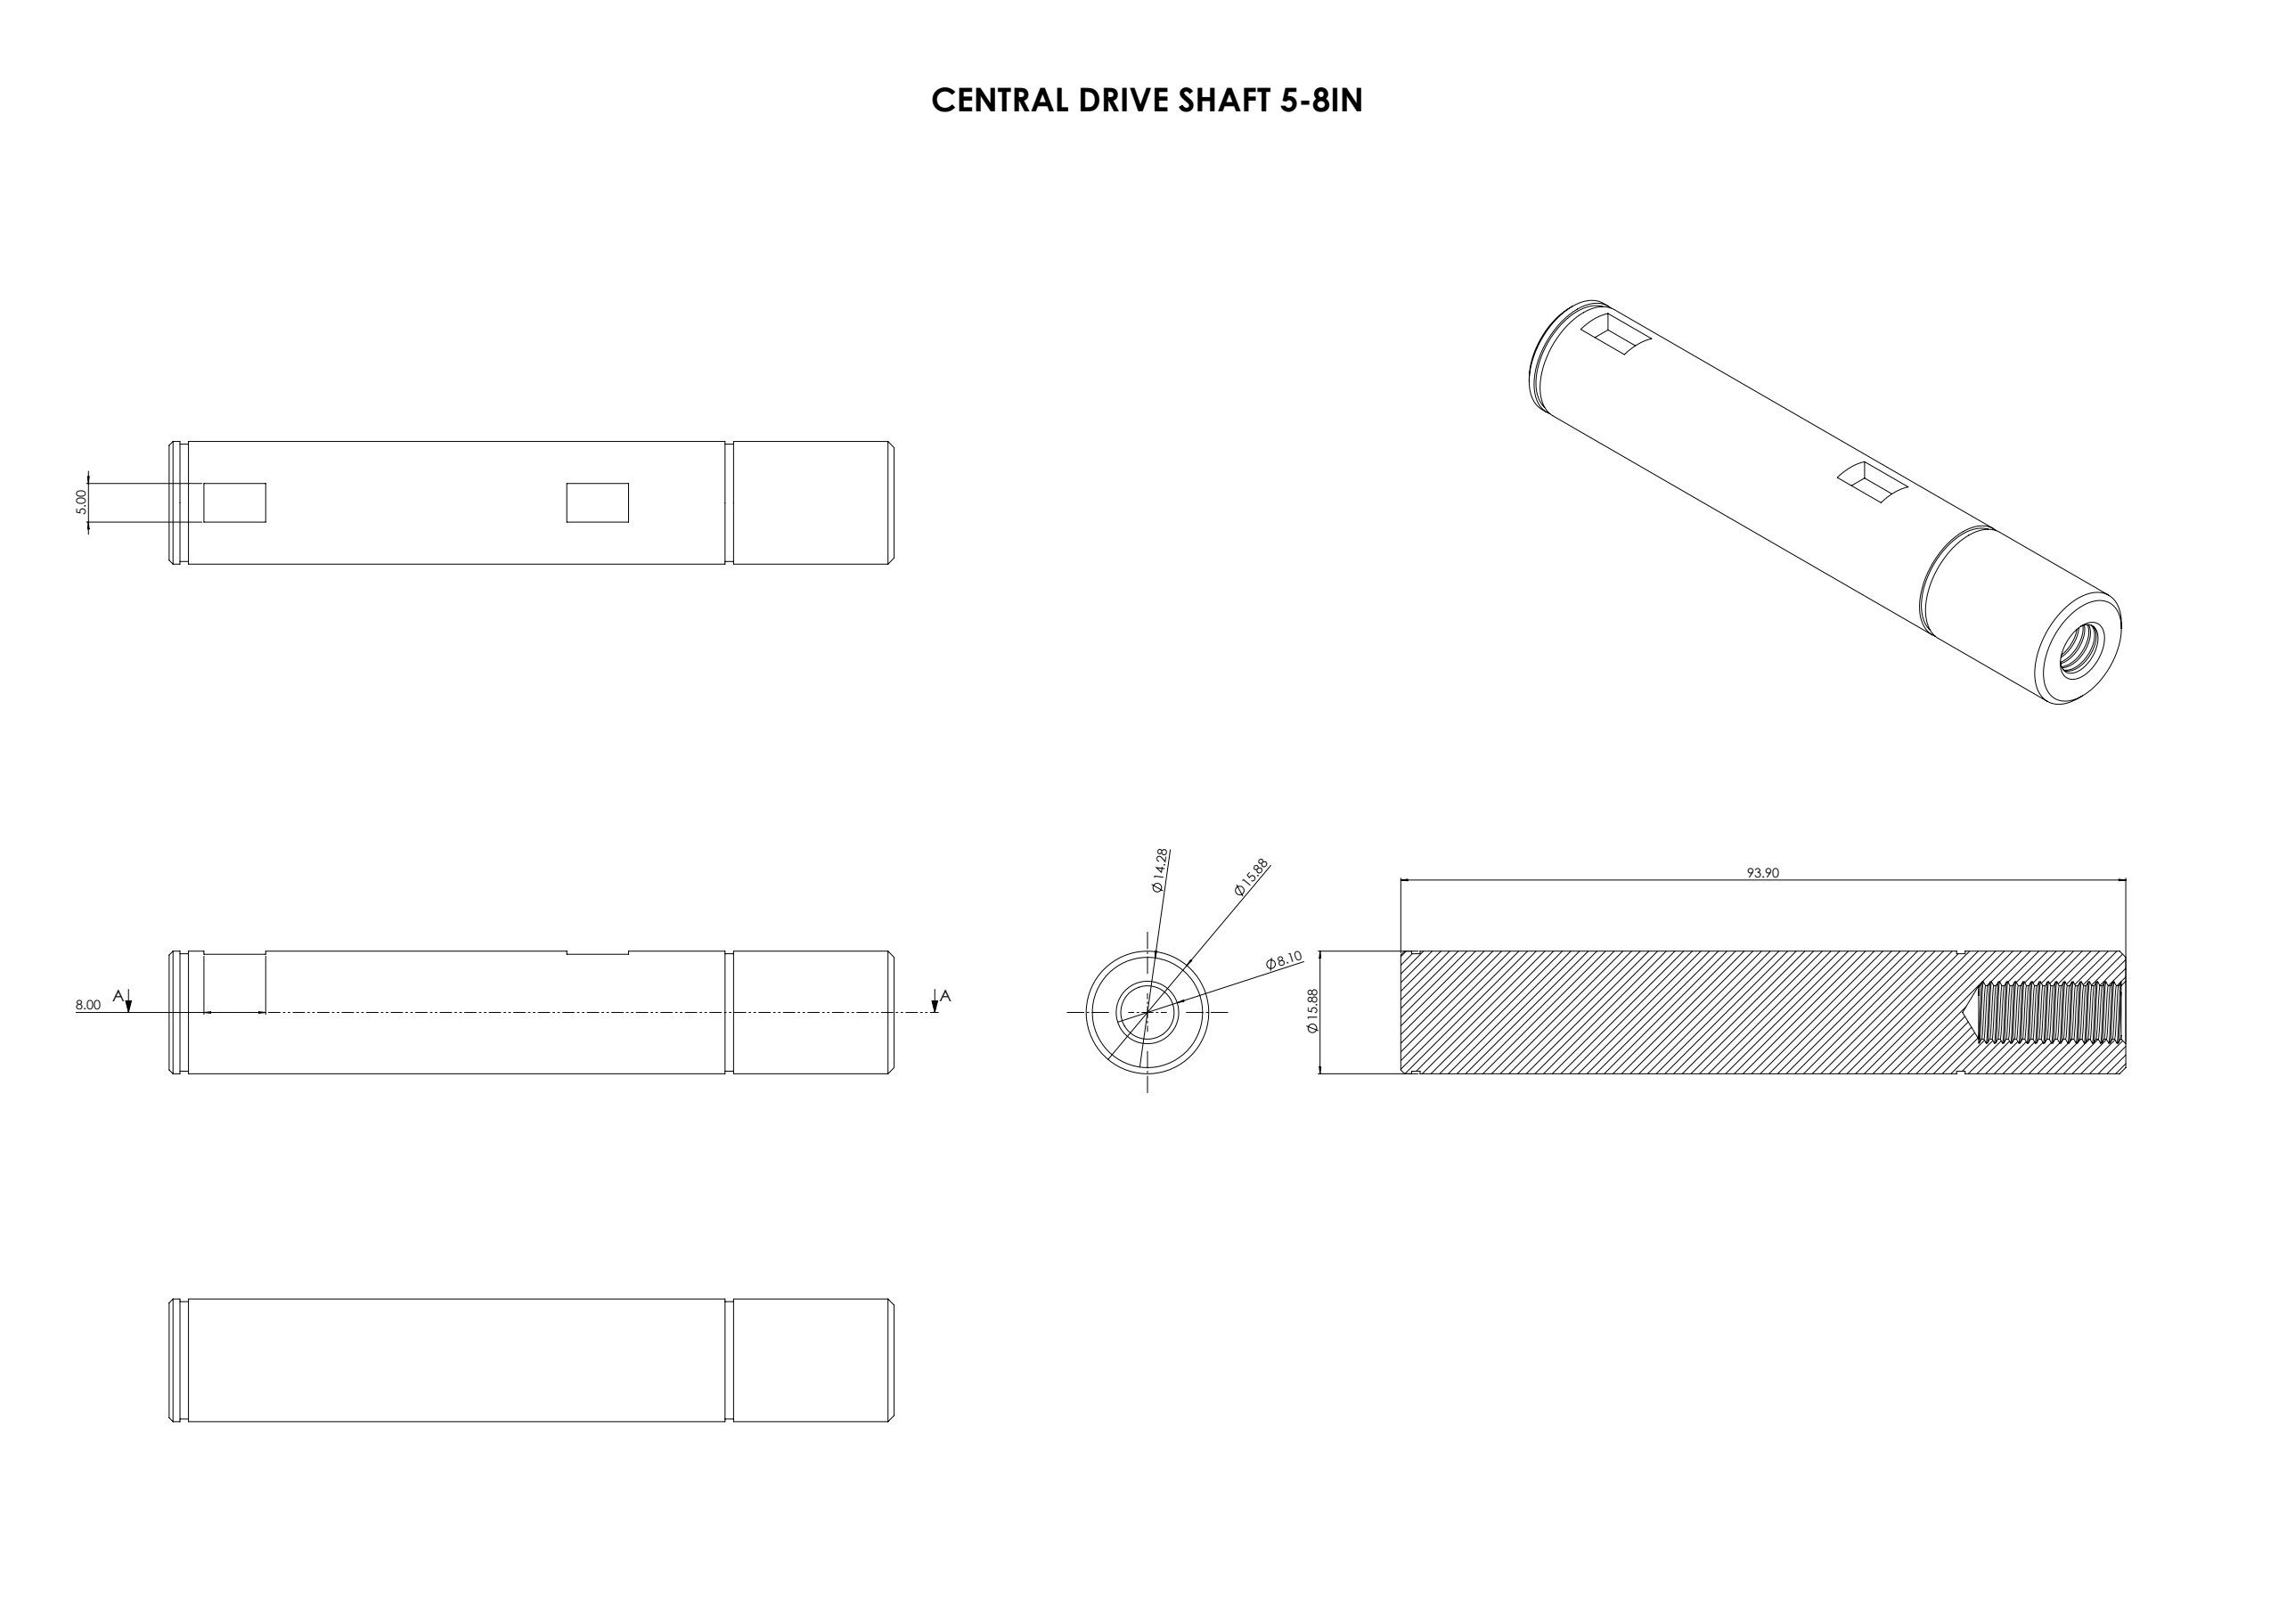
ISO-10303-21;
HEADER;
/* Generated by software containing ST-Developer
 * from STEP Tools, Inc. (www.steptools.com) 
 */

FILE_DESCRIPTION(
/* description */ (''),
/* implementation_level */ '2;1');

FILE_NAME(
/* name */ '03_Central_Drive_Shaft_5-8in.step',
/* time_stamp */ '2026-10-24T13:41:11-07:00',
/* author */ (''),
/* organization */ (''),
/* preprocessor_version */ 'ST-DEVELOPER v20.2',
/* originating_system */ 'Autodesk Translation Framework v15.15.0.0',
/* authorisation */ '');

FILE_SCHEMA (('AUTOMOTIVE_DESIGN { 1 0 10303 214 3 1 1 }'));
ENDSEC;

DATA;
#10=MECHANICAL_DESIGN_GEOMETRIC_PRESENTATION_REPRESENTATION('',(#123),#12813);
#85=CONICAL_SURFACE('',#4661,1.775,1.02974425867666);
#86=CONICAL_SURFACE('',#4663,3.85,0.785398163397459);
#87=CONICAL_SURFACE('',#4698,7.69,0.785398163397449);
#88=CONICAL_SURFACE('',#4701,7.54,0.785398163397436);
#103=SHAPE_REPRESENTATION_RELATIONSHIP('SRR','None',#12856,#113);
#113=ADVANCED_BREP_SHAPE_REPRESENTATION('',(#133),#12805);
#123=STYLED_ITEM('',(#12974),#133);
#133=MANIFOLD_SOLID_BREP('Body1',#4386);
#146=FACE_BOUND('',#701,.T.);
#147=FACE_BOUND('',#704,.T.);
#148=FACE_BOUND('',#706,.T.);
#149=FACE_BOUND('',#707,.T.);
#150=FACE_BOUND('',#709,.T.);
#151=FACE_BOUND('',#712,.T.);
#152=FACE_BOUND('',#719,.T.);
#178=PLANE('',#4654);
#179=PLANE('',#4658);
#180=PLANE('',#4665);
#181=PLANE('',#4666);
#182=PLANE('',#4668);
#183=PLANE('',#4669);
#184=PLANE('',#4671);
#185=PLANE('',#4672);
#186=PLANE('',#4673);
#187=PLANE('',#4675);
#188=PLANE('',#4676);
#189=PLANE('',#4678);
#190=PLANE('',#4679);
#191=PLANE('',#4684);
#192=PLANE('',#4688);
#193=PLANE('',#4692);
#194=PLANE('',#4696);
#195=PLANE('',#4703);
#306=B_SPLINE_SURFACE_WITH_KNOTS('',3,3,((#9182,#9183,#9184,#9185,#9186,
#9187,#9188,#9189,#9190,#9191,#9192,#9193,#9194,#9195,#9196,#9197,#9198,
#9199,#9200,#9201,#9202,#9203,#9204,#9205,#9206,#9207,#9208,#9209,#9210,
#9211,#9212,#9213,#9214,#9215,#9216,#9217,#9218,#9219,#9220,#9221,#9222,
#9223,#9224,#9225,#9226,#9227,#9228,#9229,#9230,#9231,#9232,#9233,#9234,
#9235,#9236,#9237,#9238,#9239,#9240,#9241,#9242,#9243,#9244,#9245,#9246,
#9247,#9248,#9249,#9250,#9251,#9252,#9253,#9254,#9255,#9256,#9257,#9258,
#9259,#9260,#9261,#9262,#9263,#9264,#9265,#9266,#9267,#9268,#9269,#9270,
#9271,#9272,#9273,#9274,#9275,#9276,#9277,#9278,#9279,#9280,#9281,#9282,
#9283,#9284,#9285,#9286,#9287,#9288,#9289,#9290,#9291,#9292,#9293,#9294,
#9295,#9296),(#9297,#9298,#9299,#9300,#9301,#9302,#9303,#9304,#9305,#9306,
#9307,#9308,#9309,#9310,#9311,#9312,#9313,#9314,#9315,#9316,#9317,#9318,
#9319,#9320,#9321,#9322,#9323,#9324,#9325,#9326,#9327,#9328,#9329,#9330,
#9331,#9332,#9333,#9334,#9335,#9336,#9337,#9338,#9339,#9340,#9341,#9342,
#9343,#9344,#9345,#9346,#9347,#9348,#9349,#9350,#9351,#9352,#9353,#9354,
#9355,#9356,#9357,#9358,#9359,#9360,#9361,#9362,#9363,#9364,#9365,#9366,
#9367,#9368,#9369,#9370,#9371,#9372,#9373,#9374,#9375,#9376,#9377,#9378,
#9379,#9380,#9381,#9382,#9383,#9384,#9385,#9386,#9387,#9388,#9389,#9390,
#9391,#9392,#9393,#9394,#9395,#9396,#9397,#9398,#9399,#9400,#9401,#9402,
#9403,#9404,#9405,#9406,#9407,#9408,#9409,#9410,#9411),(#9412,#9413,#9414,
#9415,#9416,#9417,#9418,#9419,#9420,#9421,#9422,#9423,#9424,#9425,#9426,
#9427,#9428,#9429,#9430,#9431,#9432,#9433,#9434,#9435,#9436,#9437,#9438,
#9439,#9440,#9441,#9442,#9443,#9444,#9445,#9446,#9447,#9448,#9449,#9450,
#9451,#9452,#9453,#9454,#9455,#9456,#9457,#9458,#9459,#9460,#9461,#9462,
#9463,#9464,#9465,#9466,#9467,#9468,#9469,#9470,#9471,#9472,#9473,#9474,
#9475,#9476,#9477,#9478,#9479,#9480,#9481,#9482,#9483,#9484,#9485,#9486,
#9487,#9488,#9489,#9490,#9491,#9492,#9493,#9494,#9495,#9496,#9497,#9498,
#9499,#9500,#9501,#9502,#9503,#9504,#9505,#9506,#9507,#9508,#9509,#9510,
#9511,#9512,#9513,#9514,#9515,#9516,#9517,#9518,#9519,#9520,#9521,#9522,
#9523,#9524,#9525,#9526),(#9527,#9528,#9529,#9530,#9531,#9532,#9533,#9534,
#9535,#9536,#9537,#9538,#9539,#9540,#9541,#9542,#9543,#9544,#9545,#9546,
#9547,#9548,#9549,#9550,#9551,#9552,#9553,#9554,#9555,#9556,#9557,#9558,
#9559,#9560,#9561,#9562,#9563,#9564,#9565,#9566,#9567,#9568,#9569,#9570,
#9571,#9572,#9573,#9574,#9575,#9576,#9577,#9578,#9579,#9580,#9581,#9582,
#9583,#9584,#9585,#9586,#9587,#9588,#9589,#9590,#9591,#9592,#9593,#9594,
#9595,#9596,#9597,#9598,#9599,#9600,#9601,#9602,#9603,#9604,#9605,#9606,
#9607,#9608,#9609,#9610,#9611,#9612,#9613,#9614,#9615,#9616,#9617,#9618,
#9619,#9620,#9621,#9622,#9623,#9624,#9625,#9626,#9627,#9628,#9629,#9630,
#9631,#9632,#9633,#9634,#9635,#9636,#9637,#9638,#9639,#9640,#9641)),
 .UNSPECIFIED.,.F.,.F.,.F.,(4,4),(4,1,1,1,1,1,1,1,1,1,1,1,1,1,1,1,1,1,1,
1,1,1,1,1,1,1,1,1,1,1,1,1,1,1,1,1,1,1,1,1,1,1,1,1,1,1,1,1,1,1,1,1,1,1,1,
1,1,1,1,1,1,1,1,1,1,1,1,1,1,1,1,1,1,1,1,1,1,1,1,1,1,1,1,1,1,1,1,1,1,1,1,
1,1,1,1,1,1,1,1,1,1,1,1,1,1,1,1,1,1,1,1,1,4),(0.,0.0593920221915367),(11.8785778954414,
12.8729398037614,13.8673017120813,14.8616636204013,15.8560255287213,16.8503874370412,
17.8447493453612,18.8391112536811,19.8334731620011,20.8278350703211,21.822196978641,
22.816558886961,23.810920795281,24.8052827036009,25.7996446119209,26.7940065202408,
27.7883684285608,28.7827303368808,29.7770922452007,30.7714541535207,31.7658160618407,
32.7601779701606,33.7545398784806,34.7489017868006,35.7432636951205,36.7376256034405,
37.7319875117605,38.7263494200804,39.7207113284004,40.7150732367203,41.7094351450403,
42.7037970533603,43.6981589616802,44.6925208700002,45.6868827783202,46.6812446866401,
47.6756065949601,48.6699685032801,49.6643304116,50.65869231992,51.6530542282399,
52.6474161365599,53.6417780448799,54.6361399531998,55.6305018615198,56.6248637698398,
57.6192256781597,58.6135875864797,59.6079494947996,60.6023114031196,61.5966733114396,
62.5910352197595,63.5853971280795,64.5797590363995,65.5741209447194,66.5684828530394,
67.5628447613594,68.5572066696793,69.5515685779993,70.5459304863193,71.5402923946392,
72.5346543029592,73.5290162112791,74.5233781195991,75.5177400279191,76.512101936239,
77.506463844559,78.500825752879,79.4951876611989,80.4895495695189,81.4839114778388,
82.4782733861588,83.4726352944788,84.4669972027987,85.4613591111187,86.4557210194387,
87.4500829277586,88.4444448360786,89.4388067443986,90.4331686527185,91.4275305610385,
92.4218924693585,93.4162543776784,94.4106162859984,95.4049781943183,96.3993401026383,
97.3937020109583,98.3880639192782,99.3824258275982,100.376787735918,101.371149644238,
102.365511552558,103.359873460878,104.354235369198,105.348597277518,106.342959185838,
107.337321094158,108.331683002478,109.326044910798,110.320406819118,111.314768727438,
112.309130635758,113.303492544078,114.297854452398,115.292216360718,116.286578269038,
117.280940177358,118.275302085678,119.269663993997,120.264025902317,121.258387810637,
122.252749718957,123.247111627277),.UNSPECIFIED.);
#307=B_SPLINE_SURFACE_WITH_KNOTS('',3,3,((#9835,#9836,#9837,#9838,#9839,
#9840,#9841,#9842,#9843,#9844,#9845,#9846,#9847,#9848,#9849,#9850,#9851,
#9852,#9853,#9854,#9855,#9856,#9857,#9858,#9859,#9860,#9861,#9862,#9863,
#9864,#9865,#9866,#9867,#9868,#9869,#9870,#9871,#9872,#9873,#9874,#9875,
#9876,#9877,#9878,#9879,#9880,#9881,#9882,#9883,#9884,#9885,#9886,#9887,
#9888,#9889,#9890,#9891,#9892,#9893,#9894,#9895,#9896,#9897,#9898,#9899,
#9900,#9901,#9902,#9903,#9904,#9905,#9906,#9907,#9908,#9909,#9910,#9911,
#9912,#9913,#9914,#9915,#9916,#9917,#9918,#9919,#9920,#9921,#9922,#9923,
#9924,#9925,#9926,#9927,#9928,#9929,#9930,#9931,#9932,#9933,#9934,#9935,
#9936,#9937,#9938,#9939,#9940,#9941,#9942,#9943,#9944,#9945,#9946,#9947,
#9948,#9949),(#9950,#9951,#9952,#9953,#9954,#9955,#9956,#9957,#9958,#9959,
#9960,#9961,#9962,#9963,#9964,#9965,#9966,#9967,#9968,#9969,#9970,#9971,
#9972,#9973,#9974,#9975,#9976,#9977,#9978,#9979,#9980,#9981,#9982,#9983,
#9984,#9985,#9986,#9987,#9988,#9989,#9990,#9991,#9992,#9993,#9994,#9995,
#9996,#9997,#9998,#9999,#10000,#10001,#10002,#10003,#10004,#10005,#10006,
#10007,#10008,#10009,#10010,#10011,#10012,#10013,#10014,#10015,#10016,#10017,
#10018,#10019,#10020,#10021,#10022,#10023,#10024,#10025,#10026,#10027,#10028,
#10029,#10030,#10031,#10032,#10033,#10034,#10035,#10036,#10037,#10038,#10039,
#10040,#10041,#10042,#10043,#10044,#10045,#10046,#10047,#10048,#10049,#10050,
#10051,#10052,#10053,#10054,#10055,#10056,#10057,#10058,#10059,#10060,#10061,
#10062,#10063,#10064),(#10065,#10066,#10067,#10068,#10069,#10070,#10071,
#10072,#10073,#10074,#10075,#10076,#10077,#10078,#10079,#10080,#10081,#10082,
#10083,#10084,#10085,#10086,#10087,#10088,#10089,#10090,#10091,#10092,#10093,
#10094,#10095,#10096,#10097,#10098,#10099,#10100,#10101,#10102,#10103,#10104,
#10105,#10106,#10107,#10108,#10109,#10110,#10111,#10112,#10113,#10114,#10115,
#10116,#10117,#10118,#10119,#10120,#10121,#10122,#10123,#10124,#10125,#10126,
#10127,#10128,#10129,#10130,#10131,#10132,#10133,#10134,#10135,#10136,#10137,
#10138,#10139,#10140,#10141,#10142,#10143,#10144,#10145,#10146,#10147,#10148,
#10149,#10150,#10151,#10152,#10153,#10154,#10155,#10156,#10157,#10158,#10159,
#10160,#10161,#10162,#10163,#10164,#10165,#10166,#10167,#10168,#10169,#10170,
#10171,#10172,#10173,#10174,#10175,#10176,#10177,#10178,#10179),(#10180,
#10181,#10182,#10183,#10184,#10185,#10186,#10187,#10188,#10189,#10190,#10191,
#10192,#10193,#10194,#10195,#10196,#10197,#10198,#10199,#10200,#10201,#10202,
#10203,#10204,#10205,#10206,#10207,#10208,#10209,#10210,#10211,#10212,#10213,
#10214,#10215,#10216,#10217,#10218,#10219,#10220,#10221,#10222,#10223,#10224,
#10225,#10226,#10227,#10228,#10229,#10230,#10231,#10232,#10233,#10234,#10235,
#10236,#10237,#10238,#10239,#10240,#10241,#10242,#10243,#10244,#10245,#10246,
#10247,#10248,#10249,#10250,#10251,#10252,#10253,#10254,#10255,#10256,#10257,
#10258,#10259,#10260,#10261,#10262,#10263,#10264,#10265,#10266,#10267,#10268,
#10269,#10270,#10271,#10272,#10273,#10274,#10275,#10276,#10277,#10278,#10279,
#10280,#10281,#10282,#10283,#10284,#10285,#10286,#10287,#10288,#10289,#10290,
#10291,#10292,#10293,#10294)),.UNSPECIFIED.,.F.,.F.,.F.,(4,4),(4,1,1,1,
1,1,1,1,1,1,1,1,1,1,1,1,1,1,1,1,1,1,1,1,1,1,1,1,1,1,1,1,1,1,1,1,1,1,1,1,
1,1,1,1,1,1,1,1,1,1,1,1,1,1,1,1,1,1,1,1,1,1,1,1,1,1,1,1,1,1,1,1,1,1,1,1,
1,1,1,1,1,1,1,1,1,1,1,1,1,1,1,1,1,1,1,1,1,1,1,1,1,1,1,1,1,1,1,1,1,1,1,1,
4),(0.,0.0593920221915367),(14.6327430048308,15.6271049131507,16.6214668214707,
17.6158287297907,18.6101906381106,19.6045525464306,20.5989144547506,21.5932763630705,
22.5876382713905,23.5820001797105,24.5763620880304,25.5707239963504,26.5650859046703,
27.5594478129903,28.5538097213103,29.5481716296302,30.5425335379502,31.5368954462702,
32.5312573545901,33.5256192629101,34.5199811712301,35.51434307955,36.50870498787,
37.5030668961899,38.4974288045099,39.4917907128299,40.4861526211498,41.4805145294698,
42.4748764377898,43.4692383461097,44.4636002544297,45.4579621627497,46.4523240710696,
47.4466859793896,48.4410478877095,49.4354097960295,50.4297717043495,51.4241336126694,
52.4184955209894,53.4128574293094,54.4072193376293,55.4015812459493,56.3959431542693,
57.3903050625892,58.3846669709092,59.3790288792291,60.3733907875491,61.3677526958691,
62.362114604189,63.356476512509,64.350838420829,65.3452003291489,66.3395622374689,
67.3339241457888,68.3282860541088,69.3226479624288,70.3170098707487,71.3113717790687,
72.3057336873887,73.3000955957086,74.2944575040286,75.2888194123486,76.2831813206685,
77.2775432289885,78.2719051373085,79.2662670456284,80.2606289539484,81.2549908622683,
82.2493527705883,83.2437146789083,84.2380765872282,85.2324384955482,86.2268004038682,
87.2211623121881,88.2155242205081,89.209886128828,90.204248037148,91.198609945468,
92.1929718537879,93.1873337621079,94.1816956704279,95.1760575787478,96.1704194870678,
97.1647813953878,98.1591433037077,99.1535052120277,100.147867120348,101.142229028668,
102.136590936988,103.130952845308,104.125314753628,105.119676661947,106.114038570267,
107.108400478587,108.102762386907,109.097124295227,110.091486203547,111.085848111867,
112.080210020187,113.074571928507,114.068933836827,115.063295745147,116.057657653467,
117.052019561787,118.046381470107,119.040743378427,120.035105286747,121.029467195067,
122.023829103387,123.018191011707,124.012552920027,125.006914828347,126.001276736667),
 .UNSPECIFIED.);
#372=FACE_OUTER_BOUND('',#647,.T.);
#373=FACE_OUTER_BOUND('',#648,.T.);
#374=FACE_OUTER_BOUND('',#649,.T.);
#375=FACE_OUTER_BOUND('',#650,.T.);
#376=FACE_OUTER_BOUND('',#651,.T.);
#377=FACE_OUTER_BOUND('',#652,.T.);
#378=FACE_OUTER_BOUND('',#653,.T.);
#379=FACE_OUTER_BOUND('',#654,.T.);
#380=FACE_OUTER_BOUND('',#655,.T.);
#381=FACE_OUTER_BOUND('',#656,.T.);
#382=FACE_OUTER_BOUND('',#657,.T.);
#383=FACE_OUTER_BOUND('',#658,.T.);
#384=FACE_OUTER_BOUND('',#659,.T.);
#385=FACE_OUTER_BOUND('',#660,.T.);
#386=FACE_OUTER_BOUND('',#661,.T.);
#387=FACE_OUTER_BOUND('',#662,.T.);
#388=FACE_OUTER_BOUND('',#663,.T.);
#389=FACE_OUTER_BOUND('',#664,.T.);
#390=FACE_OUTER_BOUND('',#665,.T.);
#391=FACE_OUTER_BOUND('',#666,.T.);
#392=FACE_OUTER_BOUND('',#667,.T.);
#393=FACE_OUTER_BOUND('',#668,.T.);
#394=FACE_OUTER_BOUND('',#669,.T.);
#395=FACE_OUTER_BOUND('',#670,.T.);
#396=FACE_OUTER_BOUND('',#671,.T.);
#397=FACE_OUTER_BOUND('',#672,.T.);
#398=FACE_OUTER_BOUND('',#673,.T.);
#399=FACE_OUTER_BOUND('',#674,.T.);
#400=FACE_OUTER_BOUND('',#675,.T.);
#401=FACE_OUTER_BOUND('',#676,.T.);
#402=FACE_OUTER_BOUND('',#677,.T.);
#403=FACE_OUTER_BOUND('',#678,.T.);
#404=FACE_OUTER_BOUND('',#679,.T.);
#405=FACE_OUTER_BOUND('',#680,.T.);
#406=FACE_OUTER_BOUND('',#681,.T.);
#407=FACE_OUTER_BOUND('',#682,.T.);
#408=FACE_OUTER_BOUND('',#683,.T.);
#409=FACE_OUTER_BOUND('',#684,.T.);
#410=FACE_OUTER_BOUND('',#685,.T.);
#411=FACE_OUTER_BOUND('',#686,.T.);
#412=FACE_OUTER_BOUND('',#687,.T.);
#413=FACE_OUTER_BOUND('',#688,.T.);
#414=FACE_OUTER_BOUND('',#689,.T.);
#415=FACE_OUTER_BOUND('',#690,.T.);
#416=FACE_OUTER_BOUND('',#691,.T.);
#417=FACE_OUTER_BOUND('',#692,.T.);
#418=FACE_OUTER_BOUND('',#693,.T.);
#419=FACE_OUTER_BOUND('',#694,.T.);
#420=FACE_OUTER_BOUND('',#695,.T.);
#421=FACE_OUTER_BOUND('',#696,.T.);
#422=FACE_OUTER_BOUND('',#697,.T.);
#423=FACE_OUTER_BOUND('',#698,.T.);
#424=FACE_OUTER_BOUND('',#699,.T.);
#425=FACE_OUTER_BOUND('',#700,.T.);
#426=FACE_OUTER_BOUND('',#702,.T.);
#427=FACE_OUTER_BOUND('',#703,.T.);
#428=FACE_OUTER_BOUND('',#705,.T.);
#429=FACE_OUTER_BOUND('',#708,.T.);
#430=FACE_OUTER_BOUND('',#710,.T.);
#431=FACE_OUTER_BOUND('',#711,.T.);
#432=FACE_OUTER_BOUND('',#713,.T.);
#433=FACE_OUTER_BOUND('',#714,.T.);
#434=FACE_OUTER_BOUND('',#715,.T.);
#435=FACE_OUTER_BOUND('',#716,.T.);
#436=FACE_OUTER_BOUND('',#717,.T.);
#437=FACE_OUTER_BOUND('',#718,.T.);
#647=EDGE_LOOP('',(#2997,#2998,#2999,#3000));
#648=EDGE_LOOP('',(#3001,#3002,#3003,#3004));
#649=EDGE_LOOP('',(#3005,#3006,#3007,#3008));
#650=EDGE_LOOP('',(#3009,#3010,#3011,#3012));
#651=EDGE_LOOP('',(#3013,#3014,#3015,#3016));
#652=EDGE_LOOP('',(#3017,#3018,#3019,#3020));
#653=EDGE_LOOP('',(#3021,#3022,#3023,#3024));
#654=EDGE_LOOP('',(#3025,#3026,#3027,#3028));
#655=EDGE_LOOP('',(#3029,#3030,#3031,#3032));
#656=EDGE_LOOP('',(#3033,#3034,#3035,#3036));
#657=EDGE_LOOP('',(#3037,#3038,#3039,#3040));
#658=EDGE_LOOP('',(#3041,#3042,#3043,#3044));
#659=EDGE_LOOP('',(#3045,#3046,#3047,#3048));
#660=EDGE_LOOP('',(#3049,#3050,#3051,#3052));
#661=EDGE_LOOP('',(#3053,#3054,#3055,#3056));
#662=EDGE_LOOP('',(#3057,#3058,#3059,#3060));
#663=EDGE_LOOP('',(#3061,#3062,#3063,#3064));
#664=EDGE_LOOP('',(#3065,#3066,#3067,#3068));
#665=EDGE_LOOP('',(#3069,#3070,#3071,#3072));
#666=EDGE_LOOP('',(#3073,#3074,#3075,#3076));
#667=EDGE_LOOP('',(#3077,#3078,#3079,#3080));
#668=EDGE_LOOP('',(#3081,#3082,#3083,#3084));
#669=EDGE_LOOP('',(#3085,#3086,#3087,#3088));
#670=EDGE_LOOP('',(#3089,#3090,#3091,#3092));
#671=EDGE_LOOP('',(#3093,#3094,#3095,#3096));
#672=EDGE_LOOP('',(#3097,#3098,#3099,#3100));
#673=EDGE_LOOP('',(#3101,#3102,#3103,#3104));
#674=EDGE_LOOP('',(#3105,#3106,#3107,#3108));
#675=EDGE_LOOP('',(#3109,#3110,#3111,#3112));
#676=EDGE_LOOP('',(#3113,#3114,#3115,#3116));
#677=EDGE_LOOP('',(#3117,#3118,#3119,#3120));
#678=EDGE_LOOP('',(#3121,#3122,#3123,#3124));
#679=EDGE_LOOP('',(#3125,#3126,#3127,#3128));
#680=EDGE_LOOP('',(#3129,#3130,#3131,#3132));
#681=EDGE_LOOP('',(#3133,#3134,#3135,#3136));
#682=EDGE_LOOP('',(#3137,#3138,#3139,#3140,#3141));
#683=EDGE_LOOP('',(#3142,#3143,#3144,#3145));
#684=EDGE_LOOP('',(#3146,#3147,#3148,#3149,#3150,#3151,#3152,#3153,#3154,
#3155,#3156,#3157,#3158,#3159,#3160,#3161,#3162,#3163,#3164,#3165,#3166,
#3167,#3168,#3169,#3170,#3171,#3172,#3173,#3174,#3175,#3176,#3177,#3178,
#3179,#3180,#3181,#3182,#3183,#3184));
#685=EDGE_LOOP('',(#3185,#3186,#3187,#3188,#3189));
#686=EDGE_LOOP('',(#3190,#3191,#3192,#3193,#3194,#3195,#3196,#3197,#3198,
#3199,#3200,#3201,#3202,#3203,#3204,#3205,#3206,#3207,#3208,#3209,#3210,
#3211,#3212,#3213,#3214,#3215,#3216,#3217,#3218,#3219,#3220,#3221,#3222,
#3223,#3224,#3225,#3226,#3227,#3228));
#687=EDGE_LOOP('',(#3229,#3230,#3231,#3232,#3233));
#688=EDGE_LOOP('',(#3234,#3235,#3236,#3237));
#689=EDGE_LOOP('',(#3238,#3239,#3240,#3241,#3242,#3243));
#690=EDGE_LOOP('',(#3244,#3245,#3246,#3247));
#691=EDGE_LOOP('',(#3248,#3249,#3250,#3251));
#692=EDGE_LOOP('',(#3252,#3253,#3254,#3255));
#693=EDGE_LOOP('',(#3256,#3257,#3258,#3259));
#694=EDGE_LOOP('',(#3260,#3261,#3262,#3263));
#695=EDGE_LOOP('',(#3264,#3265,#3266,#3267));
#696=EDGE_LOOP('',(#3268,#3269,#3270,#3271));
#697=EDGE_LOOP('',(#3272,#3273,#3274,#3275));
#698=EDGE_LOOP('',(#3276,#3277,#3278,#3279));
#699=EDGE_LOOP('',(#3280,#3281,#3282,#3283));
#700=EDGE_LOOP('',(#3284));
#701=EDGE_LOOP('',(#3285));
#702=EDGE_LOOP('',(#3286,#3287,#3288,#3289));
#703=EDGE_LOOP('',(#3290));
#704=EDGE_LOOP('',(#3291));
#705=EDGE_LOOP('',(#3292,#3293,#3294,#3295));
#706=EDGE_LOOP('',(#3296,#3297,#3298,#3299));
#707=EDGE_LOOP('',(#3300,#3301,#3302,#3303));
#708=EDGE_LOOP('',(#3304));
#709=EDGE_LOOP('',(#3305));
#710=EDGE_LOOP('',(#3306,#3307,#3308,#3309));
#711=EDGE_LOOP('',(#3310));
#712=EDGE_LOOP('',(#3311));
#713=EDGE_LOOP('',(#3312,#3313,#3314,#3315));
#714=EDGE_LOOP('',(#3316));
#715=EDGE_LOOP('',(#3317,#3318,#3319,#3320));
#716=EDGE_LOOP('',(#3321,#3322,#3323,#3324));
#717=EDGE_LOOP('',(#3325,#3326,#3327,#3328));
#718=EDGE_LOOP('',(#3329));
#719=EDGE_LOOP('',(#3330));
#960=CIRCLE('',#4616,3.4544);
#961=CIRCLE('',#4633,3.4544);
#962=CIRCLE('',#4635,3.96875);
#963=CIRCLE('',#4653,3.96875);
#964=CIRCLE('',#4655,3.4544);
#965=CIRCLE('',#4656,3.4544);
#966=CIRCLE('',#4659,3.4544);
#967=CIRCLE('',#4660,3.4544);
#968=CIRCLE('',#4664,4.05000000000002);
#969=CIRCLE('',#4667,7.94);
#970=CIRCLE('',#4670,7.94);
#971=CIRCLE('',#4674,7.94);
#972=CIRCLE('',#4677,7.94);
#973=CIRCLE('',#4680,7.94);
#974=CIRCLE('',#4681,7.6);
#975=CIRCLE('',#4683,7.6);
#976=CIRCLE('',#4685,7.94);
#977=CIRCLE('',#4687,7.94);
#978=CIRCLE('',#4689,7.6);
#979=CIRCLE('',#4691,7.6);
#980=CIRCLE('',#4693,7.94);
#981=CIRCLE('',#4695,7.94);
#982=CIRCLE('',#4697,7.44);
#983=CIRCLE('',#4700,7.94);
#984=CIRCLE('',#4702,7.14);
#1145=LINE('',#7735,#1375);
#1146=LINE('',#7777,#1376);
#1147=LINE('',#7825,#1377);
#1148=LINE('',#7876,#1378);
#1149=LINE('',#7927,#1379);
#1150=LINE('',#7975,#1380);
#1151=LINE('',#8026,#1381);
#1152=LINE('',#8074,#1382);
#1153=LINE('',#8125,#1383);
#1154=LINE('',#8176,#1384);
#1155=LINE('',#8224,#1385);
#1156=LINE('',#8275,#1386);
#1157=LINE('',#8326,#1387);
#1158=LINE('',#8374,#1388);
#1159=LINE('',#8425,#1389);
#1160=LINE('',#8473,#1390);
#1161=LINE('',#8524,#1391);
#1162=LINE('',#8566,#1392);
#1163=LINE('',#8583,#1393);
#1164=LINE('',#8608,#1394);
#1165=LINE('',#8633,#1395);
#1166=LINE('',#8657,#1396);
#1167=LINE('',#8682,#1397);
#1168=LINE('',#8707,#1398);
#1169=LINE('',#8731,#1399);
#1170=LINE('',#8755,#1400);
#1171=LINE('',#8781,#1401);
#1172=LINE('',#8805,#1402);
#1173=LINE('',#8829,#1403);
#1174=LINE('',#8855,#1404);
#1175=LINE('',#8879,#1405);
#1176=LINE('',#8903,#1406);
#1177=LINE('',#8928,#1407);
#1178=LINE('',#8953,#1408);
#1179=LINE('',#8977,#1409);
#1180=LINE('',#10319,#1410);
#1181=LINE('',#10323,#1411);
#1182=LINE('',#10328,#1412);
#1183=LINE('',#10330,#1413);
#1184=LINE('',#10332,#1414);
#1185=LINE('',#10333,#1415);
#1186=LINE('',#10338,#1416);
#1187=LINE('',#10339,#1417);
#1188=LINE('',#10342,#1418);
#1189=LINE('',#10344,#1419);
#1190=LINE('',#10345,#1420);
#1191=LINE('',#10348,#1421);
#1192=LINE('',#10353,#1422);
#1193=LINE('',#10355,#1423);
#1194=LINE('',#10357,#1424);
#1195=LINE('',#10358,#1425);
#1196=LINE('',#10363,#1426);
#1197=LINE('',#10364,#1427);
#1198=LINE('',#10367,#1428);
#1199=LINE('',#10369,#1429);
#1200=LINE('',#10370,#1430);
#1201=LINE('',#10373,#1431);
#1202=LINE('',#10383,#1432);
#1203=LINE('',#10389,#1433);
#1204=LINE('',#10397,#1434);
#1205=LINE('',#10403,#1435);
#1206=LINE('',#10409,#1436);
#1207=LINE('',#10413,#1437);
#1208=LINE('',#10417,#1438);
#1375=VECTOR('',#5248,3.55);
#1376=VECTOR('',#5253,3.55);
#1377=VECTOR('',#5256,3.55);
#1378=VECTOR('',#5259,3.55);
#1379=VECTOR('',#5262,3.55);
#1380=VECTOR('',#5265,3.55);
#1381=VECTOR('',#5268,3.55);
#1382=VECTOR('',#5271,3.55);
#1383=VECTOR('',#5274,3.55);
#1384=VECTOR('',#5277,3.55);
#1385=VECTOR('',#5280,3.55);
#1386=VECTOR('',#5283,3.55);
#1387=VECTOR('',#5286,3.55);
#1388=VECTOR('',#5289,3.55);
#1389=VECTOR('',#5292,3.55);
#1390=VECTOR('',#5295,3.55);
#1391=VECTOR('',#5298,3.55);
#1392=VECTOR('',#5303,3.96875);
#1393=VECTOR('',#5308,3.96875);
#1394=VECTOR('',#5311,3.96875);
#1395=VECTOR('',#5314,3.96875);
#1396=VECTOR('',#5317,3.96875);
#1397=VECTOR('',#5320,3.96875);
#1398=VECTOR('',#5323,3.96875);
#1399=VECTOR('',#5326,3.96875);
#1400=VECTOR('',#5329,3.96875);
#1401=VECTOR('',#5332,3.96875);
#1402=VECTOR('',#5335,3.96875);
#1403=VECTOR('',#5338,3.96875);
#1404=VECTOR('',#5341,3.96875);
#1405=VECTOR('',#5344,3.96875);
#1406=VECTOR('',#5347,3.96875);
#1407=VECTOR('',#5350,3.96875);
#1408=VECTOR('',#5353,3.96875);
#1409=VECTOR('',#5356,3.96875);
#1410=VECTOR('',#5375,1.775);
#1411=VECTOR('',#5380,3.85);
#1412=VECTOR('',#5385,10.);
#1413=VECTOR('',#5386,10.);
#1414=VECTOR('',#5387,10.);
#1415=VECTOR('',#5388,10.);
#1416=VECTOR('',#5393,10.);
#1417=VECTOR('',#5394,10.);
#1418=VECTOR('',#5397,10.);
#1419=VECTOR('',#5398,10.);
#1420=VECTOR('',#5399,10.);
#1421=VECTOR('',#5404,10.);
#1422=VECTOR('',#5409,10.);
#1423=VECTOR('',#5410,10.);
#1424=VECTOR('',#5411,10.);
#1425=VECTOR('',#5412,10.);
#1426=VECTOR('',#5417,10.);
#1427=VECTOR('',#5418,10.);
#1428=VECTOR('',#5421,10.);
#1429=VECTOR('',#5422,10.);
#1430=VECTOR('',#5423,10.);
#1431=VECTOR('',#5428,10.);
#1432=VECTOR('',#5441,7.6);
#1433=VECTOR('',#5448,7.94);
#1434=VECTOR('',#5459,7.6);
#1435=VECTOR('',#5466,7.94);
#1436=VECTOR('',#5475,7.69);
#1437=VECTOR('',#5480,7.94);
#1438=VECTOR('',#5485,7.54);
#1606=B_SPLINE_CURVE_WITH_KNOTS('',3,(#7737,#7738,#7739,#7740,#7741,#7742,
#7743,#7744,#7745,#7746,#7747,#7748,#7749),.UNSPECIFIED.,.F.,.F.,(4,3,3,
3,4),(107.889370485171,108.385448006876,109.379809915196,110.374171823516,
111.368533731836),.UNSPECIFIED.);
#1607=B_SPLINE_CURVE_WITH_KNOTS('',3,(#7752,#7753,#7754,#7755,#7756,#7757,
#7758,#7759,#7760,#7761,#7762,#7763,#7764,#7765,#7766,#7767,#7768,#7769,
#7770,#7771,#7772,#7773),.UNSPECIFIED.,.F.,.F.,(4,3,3,3,3,3,3,4),(-109.6055207498,
-109.379809915196,-108.385448006876,-107.391086098556,-106.396724190236,
-105.402362281916,-104.408000373596,-104.360350287381),.UNSPECIFIED.);
#1608=B_SPLINE_CURVE_WITH_KNOTS('',3,(#7778,#7779,#7780,#7781,#7782,#7783,
#7784,#7785,#7786,#7787,#7788,#7789,#7790,#7791,#7792,#7793,#7794,#7795,
#7796,#7797,#7798,#7799),.UNSPECIFIED.,.F.,.F.,(4,3,3,3,3,3,3,4),(101.606185177992,
102.419276556956,103.413638465276,104.408000373596,105.402362281916,106.396724190236,
107.391086098556,107.889370485171),.UNSPECIFIED.);
#1609=B_SPLINE_CURVE_WITH_KNOTS('',3,(#7800,#7801,#7802,#7803,#7804,#7805,
#7806,#7807,#7808,#7809,#7810,#7811,#7812,#7813,#7814,#7815,#7816,#7817,
#7818,#7819,#7820,#7821),.UNSPECIFIED.,.F.,.F.,(4,3,3,3,3,3,3,4),(-104.360350287381,
-103.413638465276,-102.419276556956,-101.424914648636,-100.430552740316,
-99.4361908319964,-98.4418289236764,-98.0771649802013),.UNSPECIFIED.);
#1610=B_SPLINE_CURVE_WITH_KNOTS('',3,(#7826,#7827,#7828,#7829,#7830,#7831,
#7832,#7833,#7834,#7835,#7836,#7837,#7838,#7839,#7840,#7841,#7842,#7843,
#7844,#7845,#7846,#7847,#7848,#7849,#7850),.UNSPECIFIED.,.F.,.F.,(4,3,3,
3,3,3,3,3,4),(95.3229998708118,95.4587431987165,96.4531051070365,97.4474670153564,
98.4418289236764,99.4361908319964,100.430552740316,101.424914648636,101.606185177992),
 .UNSPECIFIED.);
#1611=B_SPLINE_CURVE_WITH_KNOTS('',3,(#7851,#7852,#7853,#7854,#7855,#7856,
#7857,#7858,#7859,#7860,#7861,#7862,#7863,#7864,#7865,#7866,#7867,#7868,
#7869,#7870,#7871,#7872),.UNSPECIFIED.,.F.,.F.,(4,3,3,3,3,3,3,4),(-98.0771649802013,
-97.4474670153564,-96.4531051070365,-95.4587431987165,-94.4643812903965,
-93.4700193820766,-92.4756574737566,-91.7939796730218),.UNSPECIFIED.);
#1612=B_SPLINE_CURVE_WITH_KNOTS('',3,(#7877,#7878,#7879,#7880,#7881,#7882,
#7883,#7884,#7885,#7886,#7887,#7888,#7889,#7890,#7891,#7892,#7893,#7894,
#7895,#7896,#7897,#7898),.UNSPECIFIED.,.F.,.F.,(4,3,3,3,3,3,3,4),(89.0398145636323,
89.4925717487967,90.4869336571167,91.4812955654367,92.4756574737566,93.4700193820766,
94.4643812903965,95.3229998708118),.UNSPECIFIED.);
#1613=B_SPLINE_CURVE_WITH_KNOTS('',3,(#7899,#7900,#7901,#7902,#7903,#7904,
#7905,#7906,#7907,#7908,#7909,#7910,#7911,#7912,#7913,#7914,#7915,#7916,
#7917,#7918,#7919,#7920,#7921,#7922,#7923),.UNSPECIFIED.,.F.,.F.,(4,3,3,
3,3,3,3,3,4),(-91.7939796730218,-91.4812955654366,-90.4869336571167,-89.4925717487967,
-88.4982098404768,-87.5038479321568,-86.5094860238368,-85.5151241155169,
-85.5107943658422),.UNSPECIFIED.);
#1614=B_SPLINE_CURVE_WITH_KNOTS('',3,(#7928,#7929,#7930,#7931,#7932,#7933,
#7934,#7935,#7936,#7937,#7938,#7939,#7940,#7941,#7942,#7943,#7944,#7945,
#7946,#7947,#7948,#7949),.UNSPECIFIED.,.F.,.F.,(4,3,3,3,3,3,3,4),(82.7566292564527,
83.526400298877,84.5207622071969,85.5151241155169,86.5094860238368,87.5038479321568,
88.4982098404767,89.0398145636323),.UNSPECIFIED.);
#1615=B_SPLINE_CURVE_WITH_KNOTS('',3,(#7950,#7951,#7952,#7953,#7954,#7955,
#7956,#7957,#7958,#7959,#7960,#7961,#7962,#7963,#7964,#7965,#7966,#7967,
#7968,#7969,#7970,#7971),.UNSPECIFIED.,.F.,.F.,(4,3,3,3,3,3,3,4),(-85.5107943658422,
-84.5207622071969,-83.526400298877,-82.532038390557,-81.537676482237,-80.5433145739171,
-79.5489526655971,-79.2276090586625),.UNSPECIFIED.);
#1616=B_SPLINE_CURVE_WITH_KNOTS('',3,(#7976,#7977,#7978,#7979,#7980,#7981,
#7982,#7983,#7984,#7985,#7986,#7987,#7988,#7989,#7990,#7991,#7992,#7993,
#7994,#7995,#7996,#7997,#7998,#7999,#8000),.UNSPECIFIED.,.F.,.F.,(4,3,3,
3,3,3,3,3,4),(76.473443949273,76.5658669406372,77.5602288489572,78.5545907572771,
79.5489526655971,80.543314573917,81.537676482237,82.532038390557,82.7566292564527),
 .UNSPECIFIED.);
#1617=B_SPLINE_CURVE_WITH_KNOTS('',3,(#8001,#8002,#8003,#8004,#8005,#8006,
#8007,#8008,#8009,#8010,#8011,#8012,#8013,#8014,#8015,#8016,#8017,#8018,
#8019,#8020,#8021,#8022),.UNSPECIFIED.,.F.,.F.,(4,3,3,3,3,3,3,4),(-79.2276090586625,
-78.5545907572771,-77.5602288489572,-76.5658669406372,-75.5715050323172,
-74.5771431239973,-73.5827812156773,-72.944423751483),.UNSPECIFIED.);
#1618=B_SPLINE_CURVE_WITH_KNOTS('',3,(#8027,#8028,#8029,#8030,#8031,#8032,
#8033,#8034,#8035,#8036,#8037,#8038,#8039,#8040,#8041,#8042,#8043,#8044,
#8045,#8046,#8047,#8048),.UNSPECIFIED.,.F.,.F.,(4,3,3,3,3,3,3,4),(70.1902586420935,
70.5996954907174,71.5940573990374,72.5884193073573,73.5827812156773,74.5771431239973,
75.5715050323172,76.473443949273),.UNSPECIFIED.);
#1619=B_SPLINE_CURVE_WITH_KNOTS('',3,(#8049,#8050,#8051,#8052,#8053,#8054,
#8055,#8056,#8057,#8058,#8059,#8060,#8061,#8062,#8063,#8064,#8065,#8066,
#8067,#8068,#8069,#8070),.UNSPECIFIED.,.F.,.F.,(4,3,3,3,3,3,3,4),(-72.944423751483,
-72.5884193073574,-71.5940573990374,-70.5996954907174,-69.6053335823975,
-68.6109716740775,-67.6166097657575,-66.6612384443034),.UNSPECIFIED.);
#1620=B_SPLINE_CURVE_WITH_KNOTS('',3,(#8075,#8076,#8077,#8078,#8079,#8080,
#8081,#8082,#8083,#8084,#8085,#8086,#8087,#8088,#8089,#8090,#8091,#8092,
#8093,#8094,#8095,#8096),.UNSPECIFIED.,.F.,.F.,(4,3,3,3,3,3,3,4),(63.9070733349139,
64.6335240407976,65.6278859491176,66.6222478574375,67.6166097657575,68.6109716740775,
69.6053335823974,70.1902586420935),.UNSPECIFIED.);
#1621=B_SPLINE_CURVE_WITH_KNOTS('',3,(#8097,#8098,#8099,#8100,#8101,#8102,
#8103,#8104,#8105,#8106,#8107,#8108,#8109,#8110,#8111,#8112,#8113,#8114,
#8115,#8116,#8117,#8118,#8119,#8120,#8121),.UNSPECIFIED.,.F.,.F.,(4,3,3,
3,3,3,3,3,4),(-66.6612384443034,-66.6222478574376,-65.6278859491176,-64.6335240407977,
-63.6391621324777,-62.6448002241577,-61.6504383158378,-60.6560764075178,
-60.3780531371238),.UNSPECIFIED.);
#1622=B_SPLINE_CURVE_WITH_KNOTS('',3,(#8126,#8127,#8128,#8129,#8130,#8131,
#8132,#8133,#8134,#8135,#8136,#8137,#8138,#8139,#8140,#8141,#8142,#8143,
#8144,#8145,#8146,#8147,#8148,#8149,#8150),.UNSPECIFIED.,.F.,.F.,(4,3,3,
3,3,3,3,3,4),(57.6238880277343,57.6729906825579,58.6673525908779,59.6617144991978,
60.6560764075178,61.6504383158377,62.6448002241577,63.6391621324777,63.9070733349139),
 .UNSPECIFIED.);
#1623=B_SPLINE_CURVE_WITH_KNOTS('',3,(#8151,#8152,#8153,#8154,#8155,#8156,
#8157,#8158,#8159,#8160,#8161,#8162,#8163,#8164,#8165,#8166,#8167,#8168,
#8169,#8170,#8171,#8172),.UNSPECIFIED.,.F.,.F.,(4,3,3,3,3,3,3,4),(-60.3780531371238,
-59.6617144991978,-58.6673525908779,-57.6729906825579,-56.6786287742379,
-55.684266865918,-54.689904957598,-54.0948678299441),.UNSPECIFIED.);
#1624=B_SPLINE_CURVE_WITH_KNOTS('',3,(#8177,#8178,#8179,#8180,#8181,#8182,
#8183,#8184,#8185,#8186,#8187,#8188,#8189,#8190,#8191,#8192,#8193,#8194,
#8195,#8196,#8197,#8198),.UNSPECIFIED.,.F.,.F.,(4,3,3,3,3,3,3,4),(51.3407027205547,
51.7068192326381,52.7011811409581,53.695543049278,54.689904957598,55.684266865918,
56.6786287742379,57.6238880277343),.UNSPECIFIED.);
#1625=B_SPLINE_CURVE_WITH_KNOTS('',3,(#8199,#8200,#8201,#8202,#8203,#8204,
#8205,#8206,#8207,#8208,#8209,#8210,#8211,#8212,#8213,#8214,#8215,#8216,
#8217,#8218,#8219,#8220),.UNSPECIFIED.,.F.,.F.,(4,3,3,3,3,3,3,4),(-54.0948678299441,
-53.695543049278,-52.7011811409581,-51.7068192326381,-50.7124573243181,
-49.7180954159982,-48.7237335076782,-47.8116825227646),.UNSPECIFIED.);
#1626=B_SPLINE_CURVE_WITH_KNOTS('',3,(#8225,#8226,#8227,#8228,#8229,#8230,
#8231,#8232,#8233,#8234,#8235,#8236,#8237,#8238,#8239,#8240,#8241,#8242,
#8243,#8244,#8245,#8246),.UNSPECIFIED.,.F.,.F.,(4,3,3,3,3,3,3,4),(45.0575174133751,
45.7406477827183,46.7350096910383,47.7293715993583,48.7237335076782,49.7180954159982,
50.7124573243181,51.3407027205547),.UNSPECIFIED.);
#1627=B_SPLINE_CURVE_WITH_KNOTS('',3,(#8247,#8248,#8249,#8250,#8251,#8252,
#8253,#8254,#8255,#8256,#8257,#8258,#8259,#8260,#8261,#8262,#8263,#8264,
#8265,#8266,#8267,#8268,#8269,#8270,#8271),.UNSPECIFIED.,.F.,.F.,(4,3,3,
3,3,3,3,3,4),(-47.8116825227646,-47.7293715993582,-46.7350096910383,-45.7406477827183,
-44.7462858743984,-43.7519239660784,-42.7575620577584,-41.7632001494385,
-41.528497215585),.UNSPECIFIED.);
#1628=B_SPLINE_CURVE_WITH_KNOTS('',3,(#8276,#8277,#8278,#8279,#8280,#8281,
#8282,#8283,#8284,#8285,#8286,#8287,#8288,#8289,#8290,#8291,#8292,#8293,
#8294,#8295,#8296,#8297,#8298,#8299,#8300),.UNSPECIFIED.,.F.,.F.,(4,3,3,
3,3,3,3,3,4),(38.7743321061955,38.7801144244786,39.7744763327985,40.7688382411185,
41.7632001494385,42.7575620577584,43.7519239660784,44.7462858743984,45.0575174133751),
 .UNSPECIFIED.);
#1629=B_SPLINE_CURVE_WITH_KNOTS('',3,(#8301,#8302,#8303,#8304,#8305,#8306,
#8307,#8308,#8309,#8310,#8311,#8312,#8313,#8314,#8315,#8316,#8317,#8318,
#8319,#8320,#8321,#8322),.UNSPECIFIED.,.F.,.F.,(4,3,3,3,3,3,3,4),(-41.528497215585,
-40.7688382411185,-39.7744763327985,-38.7801144244786,-37.7857525161586,
-36.7913906078387,-35.7970286995187,-35.2453119084054),.UNSPECIFIED.);
#1630=B_SPLINE_CURVE_WITH_KNOTS('',3,(#8327,#8328,#8329,#8330,#8331,#8332,
#8333,#8334,#8335,#8336,#8337,#8338,#8339,#8340,#8341,#8342,#8343,#8344,
#8345,#8346,#8347,#8348),.UNSPECIFIED.,.F.,.F.,(4,3,3,3,3,3,3,4),(32.491146799016,
32.8139429745588,33.8083048828788,34.8026667911987,35.7970286995187,36.7913906078386,
37.7857525161586,38.7743321061955),.UNSPECIFIED.);
#1631=B_SPLINE_CURVE_WITH_KNOTS('',3,(#8349,#8350,#8351,#8352,#8353,#8354,
#8355,#8356,#8357,#8358,#8359,#8360,#8361,#8362,#8363,#8364,#8365,#8366,
#8367,#8368,#8369,#8370),.UNSPECIFIED.,.F.,.F.,(4,3,3,3,3,3,3,4),(-35.2453119084054,
-34.8026667911987,-33.8083048828788,-32.8139429745588,-31.8195810662388,
-30.8252191579189,-29.8308572495989,-28.9621266012258),.UNSPECIFIED.);
#1632=B_SPLINE_CURVE_WITH_KNOTS('',3,(#8375,#8376,#8377,#8378,#8379,#8380,
#8381,#8382,#8383,#8384,#8385,#8386,#8387,#8388,#8389,#8390,#8391,#8392,
#8393,#8394,#8395,#8396),.UNSPECIFIED.,.F.,.F.,(4,3,3,3,3,3,3,4),(26.2079614918363,
26.847771524639,27.842133432959,28.8364953412789,29.8308572495989,30.8252191579189,
31.8195810662388,32.491146799016),.UNSPECIFIED.);
#1633=B_SPLINE_CURVE_WITH_KNOTS('',3,(#8397,#8398,#8399,#8400,#8401,#8402,
#8403,#8404,#8405,#8406,#8407,#8408,#8409,#8410,#8411,#8412,#8413,#8414,
#8415,#8416,#8417,#8418,#8419,#8420,#8421),.UNSPECIFIED.,.F.,.F.,(4,3,3,
3,3,3,3,3,4),(-28.9621266012258,-28.836495341279,-27.842133432959,-26.847771524639,
-25.8534096163191,-24.8590477079991,-23.8646857996791,-22.8703238913592,
-22.6789412940462),.UNSPECIFIED.);
#1634=B_SPLINE_CURVE_WITH_KNOTS('',3,(#8426,#8427,#8428,#8429,#8430,#8431,
#8432,#8433,#8434,#8435,#8436,#8437,#8438,#8439,#8440,#8441,#8442,#8443,
#8444,#8445,#8446,#8447),.UNSPECIFIED.,.F.,.F.,(4,3,3,3,3,3,3,4),(19.9247761846567,
20.8816000747192,21.8759619830392,22.8703238913592,23.8646857996791,24.8590477079991,
25.8534096163191,26.2079614918363),.UNSPECIFIED.);
#1635=B_SPLINE_CURVE_WITH_KNOTS('',3,(#8448,#8449,#8450,#8451,#8452,#8453,
#8454,#8455,#8456,#8457,#8458,#8459,#8460,#8461,#8462,#8463,#8464,#8465,
#8466,#8467,#8468,#8469),.UNSPECIFIED.,.F.,.F.,(4,3,3,3,3,3,3,4),(-22.6789412940462,
-21.8759619830392,-20.8816000747192,-19.8872381663993,-18.8928762580793,
-17.8985143497593,-16.9041524414394,-16.3957559868666),.UNSPECIFIED.);
#1636=B_SPLINE_CURVE_WITH_KNOTS('',3,(#8474,#8475,#8476,#8477,#8478,#8479,
#8480,#8481,#8482,#8483,#8484,#8485,#8486,#8487,#8488,#8489,#8490,#8491,
#8492,#8493,#8494,#8495,#8496,#8497,#8498),.UNSPECIFIED.,.F.,.F.,(4,3,3,
3,3,3,3,3,4),(13.6415908774772,13.9210667164795,14.9154286247995,15.9097905331194,
16.9041524414394,17.8985143497593,18.8928762580793,19.8872381663993,19.9247761846567),
 .UNSPECIFIED.);
#1637=B_SPLINE_CURVE_WITH_KNOTS('',3,(#8499,#8500,#8501,#8502,#8503,#8504,
#8505,#8506,#8507,#8508,#8509,#8510,#8511,#8512,#8513,#8514,#8515,#8516,
#8517,#8518,#8519,#8520),.UNSPECIFIED.,.F.,.F.,(4,3,3,3,3,3,3,4),(-16.3957559868666,
-15.9097905331194,-14.9154286247995,-13.9210667164795,-12.9267048081595,
-11.9323428998396,-10.9379809915196,-10.1125706796871),.UNSPECIFIED.);
#1638=B_SPLINE_CURVE_WITH_KNOTS('',3,(#8526,#8527,#8528,#8529,#8530,#8531,
#8532,#8533,#8534,#8535,#8536,#8537,#8538),.UNSPECIFIED.,.F.,.F.,(4,3,3,
3,4),(-3.82938537250746,-2.98308572495989,-1.98872381663993,-0.994361908319963,
0.),.UNSPECIFIED.);
#1639=B_SPLINE_CURVE_WITH_KNOTS('',3,(#8541,#8542,#8543,#8544,#8545,#8546,
#8547,#8548,#8549,#8550,#8551,#8552,#8553,#8554,#8555,#8556,#8557,#8558,
#8559,#8560,#8561,#8562),.UNSPECIFIED.,.F.,.F.,(4,3,3,3,3,3,3,4),(1.76301298203565,
1.98872381663993,2.98308572495989,3.97744763327985,4.97180954159982,5.96617144991978,
6.96053335823975,7.35840557029759),.UNSPECIFIED.);
#1640=B_SPLINE_CURVE_WITH_KNOTS('',3,(#8568,#8569,#8570,#8571),
 .UNSPECIFIED.,.F.,.F.,(4,4),(122.522113490002,123.247111627277),
 .UNSPECIFIED.);
#1641=B_SPLINE_CURVE_WITH_KNOTS('',3,(#8574,#8575,#8576,#8577,#8578,#8579),
 .UNSPECIFIED.,.F.,.F.,(4,1,1,4),(122.522113490002,123.018191011707,124.012552920027,
124.238263754631),.UNSPECIFIED.);
#1642=B_SPLINE_CURVE_WITH_KNOTS('',3,(#8584,#8585,#8586,#8587,#8588,#8589,
#8590,#8591,#8592,#8593,#8594),.UNSPECIFIED.,.F.,.F.,(4,1,1,1,1,1,1,1,4),
(116.238928182822,116.286578269038,117.280940177358,118.275302085678,119.269663993997,
120.264025902317,121.258387810637,122.252749718957,122.522113490002),
 .UNSPECIFIED.);
#1643=B_SPLINE_CURVE_WITH_KNOTS('',3,(#8595,#8596,#8597,#8598,#8599,#8600,
#8601,#8602,#8603,#8604),.UNSPECIFIED.,.F.,.F.,(4,1,1,1,1,1,1,4),(116.238928182822,
117.052019561787,118.046381470107,119.040743378427,120.035105286747,121.029467195067,
122.023829103387,122.522113490002),.UNSPECIFIED.);
#1644=B_SPLINE_CURVE_WITH_KNOTS('',3,(#8609,#8610,#8611,#8612,#8613,#8614,
#8615,#8616,#8617,#8618),.UNSPECIFIED.,.F.,.F.,(4,1,1,1,1,1,1,4),(109.955742875643,
110.320406819118,111.314768727438,112.309130635758,113.303492544078,114.297854452398,
115.292216360718,116.238928182822),.UNSPECIFIED.);
#1645=B_SPLINE_CURVE_WITH_KNOTS('',3,(#8619,#8620,#8621,#8622,#8623,#8624,
#8625,#8626,#8627,#8628,#8629),.UNSPECIFIED.,.F.,.F.,(4,1,1,1,1,1,1,1,4),
(109.955742875643,110.091486203547,111.085848111867,112.080210020187,113.074571928507,
114.068933836827,115.063295745147,116.057657653467,116.238928182822),
 .UNSPECIFIED.);
#1646=B_SPLINE_CURVE_WITH_KNOTS('',3,(#8634,#8635,#8636,#8637,#8638,#8639,
#8640,#8641,#8642,#8643),.UNSPECIFIED.,.F.,.F.,(4,1,1,1,1,1,1,4),(103.672557568463,
104.354235369198,105.348597277518,106.342959185838,107.337321094158,108.331683002478,
109.326044910798,109.955742875643),.UNSPECIFIED.);
#1647=B_SPLINE_CURVE_WITH_KNOTS('',3,(#8644,#8645,#8646,#8647,#8648,#8649,
#8650,#8651,#8652,#8653),.UNSPECIFIED.,.F.,.F.,(4,1,1,1,1,1,1,4),(103.672557568463,
104.125314753628,105.119676661947,106.114038570267,107.108400478587,108.102762386907,
109.097124295227,109.955742875643),.UNSPECIFIED.);
#1648=B_SPLINE_CURVE_WITH_KNOTS('',3,(#8658,#8659,#8660,#8661,#8662,#8663,
#8664,#8665,#8666,#8667,#8668),.UNSPECIFIED.,.F.,.F.,(4,1,1,1,1,1,1,1,4),
(97.3893722612835,97.3937020109583,98.3880639192782,99.3824258275982,100.376787735918,
101.371149644238,102.365511552558,103.359873460878,103.672557568463),
 .UNSPECIFIED.);
#1649=B_SPLINE_CURVE_WITH_KNOTS('',3,(#8669,#8670,#8671,#8672,#8673,#8674,
#8675,#8676,#8677,#8678),.UNSPECIFIED.,.F.,.F.,(4,1,1,1,1,1,1,4),(97.3893722612835,
98.1591433037077,99.1535052120277,100.147867120348,101.142229028668,102.136590936988,
103.130952845308,103.672557568463),.UNSPECIFIED.);
#1650=B_SPLINE_CURVE_WITH_KNOTS('',3,(#8683,#8684,#8685,#8686,#8687,#8688,
#8689,#8690,#8691,#8692),.UNSPECIFIED.,.F.,.F.,(4,1,1,1,1,1,1,4),(91.106186954104,
91.4275305610385,92.4218924693585,93.4162543776784,94.4106162859984,95.4049781943183,
96.3993401026383,97.3893722612835),.UNSPECIFIED.);
#1651=B_SPLINE_CURVE_WITH_KNOTS('',3,(#8693,#8694,#8695,#8696,#8697,#8698,
#8699,#8700,#8701,#8702,#8703),.UNSPECIFIED.,.F.,.F.,(4,1,1,1,1,1,1,1,4),
(91.106186954104,91.198609945468,92.1929718537879,93.1873337621079,94.1816956704279,
95.1760575787478,96.1704194870678,97.1647813953878,97.3893722612835),
 .UNSPECIFIED.);
#1652=B_SPLINE_CURVE_WITH_KNOTS('',3,(#8708,#8709,#8710,#8711,#8712,#8713,
#8714,#8715,#8716,#8717),.UNSPECIFIED.,.F.,.F.,(4,1,1,1,1,1,1,4),(84.8230016469244,
85.4613591111187,86.4557210194387,87.4500829277586,88.4444448360786,89.4388067443986,
90.4331686527185,91.106186954104),.UNSPECIFIED.);
#1653=B_SPLINE_CURVE_WITH_KNOTS('',3,(#8718,#8719,#8720,#8721,#8722,#8723,
#8724,#8725,#8726,#8727),.UNSPECIFIED.,.F.,.F.,(4,1,1,1,1,1,1,4),(84.8230016469244,
85.2324384955482,86.2268004038682,87.2211623121881,88.2155242205081,89.209886128828,
90.204248037148,91.106186954104),.UNSPECIFIED.);
#1654=B_SPLINE_CURVE_WITH_KNOTS('',3,(#8732,#8733,#8734,#8735,#8736,#8737,
#8738,#8739,#8740,#8741),.UNSPECIFIED.,.F.,.F.,(4,1,1,1,1,1,1,4),(78.5398163397447,
79.4951876611989,80.4895495695189,81.4839114778388,82.4782733861588,83.4726352944788,
84.4669972027987,84.8230016469244),.UNSPECIFIED.);
#1655=B_SPLINE_CURVE_WITH_KNOTS('',3,(#8742,#8743,#8744,#8745,#8746,#8747,
#8748,#8749,#8750,#8751),.UNSPECIFIED.,.F.,.F.,(4,1,1,1,1,1,1,4),(78.5398163397447,
79.2662670456284,80.2606289539484,81.2549908622683,82.2493527705883,83.2437146789083,
84.2380765872282,84.8230016469244),.UNSPECIFIED.);
#1656=B_SPLINE_CURVE_WITH_KNOTS('',3,(#8756,#8757,#8758,#8759,#8760,#8761,
#8762,#8763,#8764,#8765,#8766),.UNSPECIFIED.,.F.,.F.,(4,1,1,1,1,1,1,1,4),
(72.2566310325652,72.5346543029592,73.5290162112791,74.5233781195991,75.5177400279191,
76.512101936239,77.506463844559,78.500825752879,78.5398163397447),
 .UNSPECIFIED.);
#1657=B_SPLINE_CURVE_WITH_KNOTS('',3,(#8767,#8768,#8769,#8770,#8771,#8772,
#8773,#8774,#8775,#8776,#8777),.UNSPECIFIED.,.F.,.F.,(4,1,1,1,1,1,1,1,4),
(72.2566310325652,72.3057336873887,73.3000955957086,74.2944575040286,75.2888194123486,
76.2831813206685,77.2775432289885,78.2719051373085,78.5398163397447),
 .UNSPECIFIED.);
#1658=B_SPLINE_CURVE_WITH_KNOTS('',3,(#8782,#8783,#8784,#8785,#8786,#8787,
#8788,#8789,#8790,#8791),.UNSPECIFIED.,.F.,.F.,(4,1,1,1,1,1,1,4),(65.9734457253856,
66.5684828530394,67.5628447613594,68.5572066696793,69.5515685779993,70.5459304863193,
71.5402923946392,72.2566310325652),.UNSPECIFIED.);
#1659=B_SPLINE_CURVE_WITH_KNOTS('',3,(#8792,#8793,#8794,#8795,#8796,#8797,
#8798,#8799,#8800,#8801),.UNSPECIFIED.,.F.,.F.,(4,1,1,1,1,1,1,4),(65.9734457253856,
66.3395622374689,67.3339241457888,68.3282860541088,69.3226479624288,70.3170098707487,
71.3113717790687,72.2566310325652),.UNSPECIFIED.);
#1660=B_SPLINE_CURVE_WITH_KNOTS('',3,(#8806,#8807,#8808,#8809,#8810,#8811,
#8812,#8813,#8814,#8815),.UNSPECIFIED.,.F.,.F.,(4,1,1,1,1,1,1,4),(59.690260418206,
60.6023114031196,61.5966733114396,62.5910352197595,63.5853971280795,64.5797590363995,
65.5741209447194,65.9734457253856),.UNSPECIFIED.);
#1661=B_SPLINE_CURVE_WITH_KNOTS('',3,(#8816,#8817,#8818,#8819,#8820,#8821,
#8822,#8823,#8824,#8825),.UNSPECIFIED.,.F.,.F.,(4,1,1,1,1,1,1,4),(59.690260418206,
60.3733907875491,61.3677526958691,62.362114604189,63.356476512509,64.350838420829,
65.3452003291489,65.9734457253856),.UNSPECIFIED.);
#1662=B_SPLINE_CURVE_WITH_KNOTS('',3,(#8830,#8831,#8832,#8833,#8834,#8835,
#8836,#8837,#8838,#8839,#8840),.UNSPECIFIED.,.F.,.F.,(4,1,1,1,1,1,1,1,4),
(53.4070751110264,53.6417780448799,54.6361399531998,55.6305018615198,56.6248637698398,
57.6192256781597,58.6135875864797,59.6079494947996,59.690260418206),
 .UNSPECIFIED.);
#1663=B_SPLINE_CURVE_WITH_KNOTS('',3,(#8841,#8842,#8843,#8844,#8845,#8846,
#8847,#8848,#8849,#8850,#8851),.UNSPECIFIED.,.F.,.F.,(4,1,1,1,1,1,1,1,4),
(53.4070751110264,53.4128574293094,54.4072193376293,55.4015812459493,56.3959431542693,
57.3903050625892,58.3846669709092,59.3790288792291,59.690260418206),
 .UNSPECIFIED.);
#1664=B_SPLINE_CURVE_WITH_KNOTS('',3,(#8856,#8857,#8858,#8859,#8860,#8861,
#8862,#8863,#8864,#8865),.UNSPECIFIED.,.F.,.F.,(4,1,1,1,1,1,1,4),(47.1238898038468,
47.6756065949601,48.6699685032801,49.6643304116,50.65869231992,51.6530542282399,
52.6474161365599,53.4070751110264),.UNSPECIFIED.);
#1665=B_SPLINE_CURVE_WITH_KNOTS('',3,(#8866,#8867,#8868,#8869,#8870,#8871,
#8872,#8873,#8874,#8875),.UNSPECIFIED.,.F.,.F.,(4,1,1,1,1,1,1,4),(47.1238898038468,
47.4466859793896,48.4410478877095,49.4354097960295,50.4297717043495,51.4241336126694,
52.4184955209894,53.4070751110264),.UNSPECIFIED.);
#1666=B_SPLINE_CURVE_WITH_KNOTS('',3,(#8880,#8881,#8882,#8883,#8884,#8885,
#8886,#8887,#8888,#8889),.UNSPECIFIED.,.F.,.F.,(4,1,1,1,1,1,1,4),(40.8407044966672,
41.7094351450403,42.7037970533603,43.6981589616802,44.6925208700002,45.6868827783202,
46.6812446866401,47.1238898038468),.UNSPECIFIED.);
#1667=B_SPLINE_CURVE_WITH_KNOTS('',3,(#8890,#8891,#8892,#8893,#8894,#8895,
#8896,#8897,#8898,#8899),.UNSPECIFIED.,.F.,.F.,(4,1,1,1,1,1,1,4),(40.8407044966672,
41.4805145294698,42.4748764377898,43.4692383461097,44.4636002544297,45.4579621627497,
46.4523240710696,47.1238898038468),.UNSPECIFIED.);
#1668=B_SPLINE_CURVE_WITH_KNOTS('',3,(#8904,#8905,#8906,#8907,#8908,#8909,
#8910,#8911,#8912,#8913,#8914),.UNSPECIFIED.,.F.,.F.,(4,1,1,1,1,1,1,1,4),
(34.5575191894876,34.7489017868006,35.7432636951205,36.7376256034405,37.7319875117605,
38.7263494200804,39.7207113284004,40.7150732367203,40.8407044966672),
 .UNSPECIFIED.);
#1669=B_SPLINE_CURVE_WITH_KNOTS('',3,(#8915,#8916,#8917,#8918,#8919,#8920,
#8921,#8922,#8923,#8924),.UNSPECIFIED.,.F.,.F.,(4,1,1,1,1,1,1,4),(34.5575191894876,
35.51434307955,36.50870498787,37.5030668961899,38.4974288045099,39.4917907128299,
40.4861526211498,40.8407044966672),.UNSPECIFIED.);
#1670=B_SPLINE_CURVE_WITH_KNOTS('',3,(#8929,#8930,#8931,#8932,#8933,#8934,
#8935,#8936,#8937,#8938),.UNSPECIFIED.,.F.,.F.,(4,1,1,1,1,1,1,4),(28.274333882308,
28.7827303368808,29.7770922452007,30.7714541535207,31.7658160618407,32.7601779701606,
33.7545398784806,34.5575191894876),.UNSPECIFIED.);
#1671=B_SPLINE_CURVE_WITH_KNOTS('',3,(#8939,#8940,#8941,#8942,#8943,#8944,
#8945,#8946,#8947,#8948,#8949),.UNSPECIFIED.,.F.,.F.,(4,1,1,1,1,1,1,1,4),
(28.274333882308,28.5538097213103,29.5481716296302,30.5425335379502,31.5368954462702,
32.5312573545901,33.5256192629101,34.5199811712301,34.5575191894876),
 .UNSPECIFIED.);
#1672=B_SPLINE_CURVE_WITH_KNOTS('',3,(#8954,#8955,#8956,#8957,#8958,#8959,
#8960,#8961,#8962,#8963),.UNSPECIFIED.,.F.,.F.,(4,1,1,1,1,1,1,4),(21.9911485751284,
22.816558886961,23.810920795281,24.8052827036009,25.7996446119209,26.7940065202408,
27.7883684285608,28.274333882308),.UNSPECIFIED.);
#1673=B_SPLINE_CURVE_WITH_KNOTS('',3,(#8964,#8965,#8966,#8967,#8968,#8969,
#8970,#8971,#8972,#8973),.UNSPECIFIED.,.F.,.F.,(4,1,1,1,1,1,1,4),(21.9911485751284,
22.5876382713905,23.5820001797105,24.5763620880304,25.5707239963504,26.5650859046703,
27.5594478129903,28.274333882308),.UNSPECIFIED.);
#1674=B_SPLINE_CURVE_WITH_KNOTS('',3,(#8979,#8980,#8981,#8982,#8983),
 .UNSPECIFIED.,.F.,.F.,(4,1,4),(14.6327430048308,15.6271049131507,15.7079632679489),
 .UNSPECIFIED.);
#1675=B_SPLINE_CURVE_WITH_KNOTS('',3,(#8986,#8987,#8988,#8989,#8990,#8991),
 .UNSPECIFIED.,.F.,.F.,(4,1,1,4),(13.6415908774771,13.8673017120813,14.8616636204013,
15.7079632679489),.UNSPECIFIED.);
#1676=B_SPLINE_CURVE_WITH_KNOTS('',3,(#8996,#8997,#8998,#8999,#9000,#9001,
#9002,#9003,#9004,#9005,#9006,#9007,#9008,#9009,#9010,#9011,#9012,#9013,
#9014,#9015,#9016,#9017,#9018,#9019,#9020,#9021,#9022,#9023,#9024,#9025,
#9026,#9027,#9028,#9029,#9030,#9031,#9032,#9033,#9034,#9035,#9036,#9037,
#9038,#9039,#9040,#9041,#9042,#9043,#9044,#9045,#9046,#9047,#9048,#9049,
#9050,#9051,#9052,#9053,#9054,#9055,#9056,#9057,#9058,#9059,#9060,#9061,
#9062,#9063,#9064,#9065,#9066,#9067,#9068,#9069,#9070,#9071,#9072,#9073,
#9074,#9075,#9076,#9077),.UNSPECIFIED.,.F.,.F.,(4,3,3,3,3,3,3,3,3,3,3,3,
3,3,3,3,3,3,3,3,3,3,3,3,3,3,3,4),(-0.659098020064273,-0.626583361418082,
-0.593277974374451,-0.55935451242369,-0.553527494448718,-0.547862782208884,
-0.513423105891954,-0.478559830537098,-0.456043474192613,-0.446497663053644,
-0.441032459037381,-0.405381589223341,-0.36977595468836,-0.334102467234791,
-0.316265723508006,-0.30668221639439,-0.301163149286353,-0.298428979781222,
-0.2643597751017,-0.228954386588656,-0.19290020592246,-0.168787680182153,
-0.157455049850378,-0.152068965805326,-0.114051724353995,-0.076872177317131,
-0.0384360886585655,0.),.UNSPECIFIED.);
#1677=B_SPLINE_CURVE_WITH_KNOTS('',3,(#9078,#9079,#9080,#9081,#9082,#9083,
#9084,#9085,#9086,#9087,#9088,#9089,#9090,#9091,#9092,#9093,#9094,#9095,
#9096,#9097,#9098,#9099,#9100,#9101,#9102,#9103,#9104,#9105,#9106,#9107,
#9108,#9109,#9110,#9111,#9112,#9113,#9114,#9115,#9116,#9117,#9118,#9119,
#9120,#9121,#9122,#9123,#9124,#9125,#9126,#9127,#9128,#9129,#9130,#9131,
#9132,#9133,#9134,#9135,#9136,#9137,#9138,#9139,#9140,#9141,#9142,#9143,
#9144,#9145,#9146,#9147,#9148,#9149,#9150,#9151,#9152,#9153,#9154,#9155,
#9156,#9157,#9158,#9159),.UNSPECIFIED.,.F.,.F.,(4,3,3,3,3,3,3,3,3,3,3,3,
3,3,3,3,3,3,3,3,3,3,3,3,3,3,3,4),(-0.657201022293968,-0.620843507912061,
-0.583812069642265,-0.545304753610891,-0.539298492849628,-0.533288478909317,
-0.49669576643024,-0.460284093722029,-0.437217774680684,-0.425131515458518,
-0.419071806367675,-0.383242240123574,-0.34808971350986,-0.311921627450565,
-0.293837584420918,-0.284384662265536,-0.278693413802068,-0.27575354139127,
-0.241284348717361,-0.206301309944578,-0.171212377127033,-0.149810829986154,
-0.13853214715148,-0.133449179146389,-0.0991640919442515,-0.0650684826066501,
-0.0318743752082536,0.),.UNSPECIFIED.);
#1678=B_SPLINE_CURVE_WITH_KNOTS('',3,(#9161,#9162,#9163,#9164,#9165,#9166,
#9167,#9168,#9169,#9170,#9171),.UNSPECIFIED.,.F.,.F.,(4,1,1,1,1,1,1,1,4),
(15.7079632679489,15.8560255287213,16.8503874370412,17.8447493453612,18.8391112536811,
19.8334731620011,20.8278350703211,21.822196978641,21.9911485751284),
 .UNSPECIFIED.);
#1679=B_SPLINE_CURVE_WITH_KNOTS('',3,(#9172,#9173,#9174,#9175,#9176,#9177,
#9178,#9179,#9180,#9181),.UNSPECIFIED.,.F.,.F.,(4,1,1,1,1,1,1,4),(15.7079632679489,
16.6214668214707,17.6158287297907,18.6101906381106,19.6045525464306,20.5989144547506,
21.5932763630705,21.9911485751284),.UNSPECIFIED.);
#1680=B_SPLINE_CURVE_WITH_KNOTS('',3,(#9642,#9643,#9644,#9645,#9646,#9647,
#9648,#9649,#9650,#9651,#9652,#9653,#9654,#9655,#9656,#9657,#9658,#9659,
#9660,#9661,#9662,#9663,#9664,#9665,#9666,#9667,#9668,#9669,#9670,#9671,
#9672,#9673,#9674,#9675,#9676,#9677,#9678,#9679,#9680,#9681,#9682,#9683,
#9684,#9685,#9686,#9687,#9688,#9689,#9690,#9691,#9692,#9693,#9694,#9695,
#9696,#9697,#9698,#9699,#9700,#9701,#9702,#9703,#9704,#9705,#9706,#9707,
#9708,#9709,#9710,#9711,#9712,#9713,#9714,#9715,#9716,#9717,#9718,#9719,
#9720,#9721,#9722,#9723),.UNSPECIFIED.,.F.,.F.,(4,3,3,3,3,3,3,3,3,3,3,3,
3,3,3,3,3,3,3,3,3,3,3,3,3,3,3,4),(-0.659098020064319,-0.626583355717508,
-0.593277963850765,-0.559354498782614,-0.553527466898513,-0.547862778460467,
-0.513423098595221,-0.478559821819824,-0.456043466564999,-0.446497640120997,
-0.441032457407506,-0.405381588000935,-0.369775954373192,-0.334102467077208,
-0.316265723429216,-0.306682216314082,-0.301163149097039,-0.298428979781224,
-0.264359779778512,-0.22895439423595,-0.192900215169359,-0.168787688273189,
-0.157455061634061,-0.152068971468546,-0.114051728601409,-0.0768721821854325,
-0.0384360910927163,0.),.UNSPECIFIED.);
#1681=B_SPLINE_CURVE_WITH_KNOTS('',3,(#9724,#9725,#9726,#9727,#9728,#9729,
#9730,#9731,#9732,#9733,#9734,#9735,#9736,#9737,#9738,#9739,#9740,#9741,
#9742,#9743,#9744,#9745,#9746,#9747,#9748),.UNSPECIFIED.,.F.,.F.,(4,3,3,
3,3,3,3,3,4),(-10.1125706796871,-9.94361908319964,-8.94925717487967,-7.95489526655971,
-6.96053335823974,-5.96617144991978,-4.97180954159982,-3.97744763327986,
-3.82938537250746),.UNSPECIFIED.);
#1682=B_SPLINE_CURVE_WITH_KNOTS('',3,(#9750,#9751,#9752,#9753,#9754,#9755,
#9756,#9757,#9758,#9759,#9760,#9761,#9762,#9763,#9764,#9765,#9766,#9767,
#9768,#9769,#9770,#9771,#9772,#9773,#9774,#9775,#9776,#9777,#9778,#9779,
#9780,#9781,#9782,#9783,#9784,#9785,#9786,#9787,#9788,#9789,#9790,#9791,
#9792,#9793,#9794,#9795,#9796,#9797,#9798,#9799,#9800,#9801,#9802,#9803,
#9804,#9805,#9806,#9807,#9808,#9809,#9810,#9811,#9812,#9813,#9814,#9815,
#9816,#9817,#9818,#9819,#9820,#9821,#9822,#9823,#9824,#9825,#9826,#9827,
#9828,#9829,#9830,#9831),.UNSPECIFIED.,.F.,.F.,(4,3,3,3,3,3,3,3,3,3,3,3,
3,3,3,3,3,3,3,3,3,3,3,3,3,3,3,4),(-0.657201022293926,-0.620843512226781,
-0.583812075977012,-0.545304759153794,-0.539298504171762,-0.533288480271845,
-0.496695767933232,-0.460284093901184,-0.437217774837445,-0.425131516019463,
-0.419071806729443,-0.3832422403949,-0.348089712058185,-0.311921626724727,
-0.293837584057999,-0.284384661973879,-0.278693413430814,-0.27575354139127,
-0.241284348717361,-0.206301309906783,-0.171212377154442,-0.149810830010137,
-0.138532146710759,-0.133449178888522,-0.0991640917928147,-0.0650684819880444,
-0.0318743724222816,0.),.UNSPECIFIED.);
#1683=B_SPLINE_CURVE_WITH_KNOTS('',3,(#10295,#10296,#10297,#10298,#10299,
#10300,#10301,#10302,#10303,#10304,#10305,#10306,#10307,#10308,#10309,#10310,
#10311,#10312,#10313,#10314,#10315,#10316),.UNSPECIFIED.,.F.,.F.,(4,3,3,
3,3,3,3,4),(7.35840557029759,7.95489526655971,8.94925717487967,9.94361908319964,
10.9379809915196,11.9323428998396,12.9267048081595,13.6415908774772),
 .UNSPECIFIED.);
#1817=VERTEX_POINT('',#7733);
#1818=VERTEX_POINT('',#7734);
#1819=VERTEX_POINT('',#7736);
#1820=VERTEX_POINT('',#7750);
#1821=VERTEX_POINT('',#7775);
#1822=VERTEX_POINT('',#7776);
#1823=VERTEX_POINT('',#7823);
#1824=VERTEX_POINT('',#7824);
#1825=VERTEX_POINT('',#7874);
#1826=VERTEX_POINT('',#7875);
#1827=VERTEX_POINT('',#7925);
#1828=VERTEX_POINT('',#7926);
#1829=VERTEX_POINT('',#7973);
#1830=VERTEX_POINT('',#7974);
#1831=VERTEX_POINT('',#8024);
#1832=VERTEX_POINT('',#8025);
#1833=VERTEX_POINT('',#8072);
#1834=VERTEX_POINT('',#8073);
#1835=VERTEX_POINT('',#8123);
#1836=VERTEX_POINT('',#8124);
#1837=VERTEX_POINT('',#8174);
#1838=VERTEX_POINT('',#8175);
#1839=VERTEX_POINT('',#8222);
#1840=VERTEX_POINT('',#8223);
#1841=VERTEX_POINT('',#8273);
#1842=VERTEX_POINT('',#8274);
#1843=VERTEX_POINT('',#8324);
#1844=VERTEX_POINT('',#8325);
#1845=VERTEX_POINT('',#8372);
#1846=VERTEX_POINT('',#8373);
#1847=VERTEX_POINT('',#8423);
#1848=VERTEX_POINT('',#8424);
#1849=VERTEX_POINT('',#8471);
#1850=VERTEX_POINT('',#8472);
#1851=VERTEX_POINT('',#8522);
#1852=VERTEX_POINT('',#8523);
#1853=VERTEX_POINT('',#8525);
#1854=VERTEX_POINT('',#8539);
#1855=VERTEX_POINT('',#8564);
#1856=VERTEX_POINT('',#8565);
#1857=VERTEX_POINT('',#8567);
#1858=VERTEX_POINT('',#8572);
#1859=VERTEX_POINT('',#8581);
#1860=VERTEX_POINT('',#8582);
#1861=VERTEX_POINT('',#8606);
#1862=VERTEX_POINT('',#8607);
#1863=VERTEX_POINT('',#8631);
#1864=VERTEX_POINT('',#8632);
#1865=VERTEX_POINT('',#8655);
#1866=VERTEX_POINT('',#8656);
#1867=VERTEX_POINT('',#8680);
#1868=VERTEX_POINT('',#8681);
#1869=VERTEX_POINT('',#8705);
#1870=VERTEX_POINT('',#8706);
#1871=VERTEX_POINT('',#8729);
#1872=VERTEX_POINT('',#8730);
#1873=VERTEX_POINT('',#8753);
#1874=VERTEX_POINT('',#8754);
#1875=VERTEX_POINT('',#8779);
#1876=VERTEX_POINT('',#8780);
#1877=VERTEX_POINT('',#8803);
#1878=VERTEX_POINT('',#8804);
#1879=VERTEX_POINT('',#8827);
#1880=VERTEX_POINT('',#8828);
#1881=VERTEX_POINT('',#8853);
#1882=VERTEX_POINT('',#8854);
#1883=VERTEX_POINT('',#8877);
#1884=VERTEX_POINT('',#8878);
#1885=VERTEX_POINT('',#8901);
#1886=VERTEX_POINT('',#8902);
#1887=VERTEX_POINT('',#8926);
#1888=VERTEX_POINT('',#8927);
#1889=VERTEX_POINT('',#8951);
#1890=VERTEX_POINT('',#8952);
#1891=VERTEX_POINT('',#8975);
#1892=VERTEX_POINT('',#8976);
#1893=VERTEX_POINT('',#8978);
#1894=VERTEX_POINT('',#8984);
#1895=VERTEX_POINT('',#8993);
#1896=VERTEX_POINT('',#9832);
#1897=VERTEX_POINT('',#10318);
#1898=VERTEX_POINT('',#10322);
#1899=VERTEX_POINT('',#10326);
#1900=VERTEX_POINT('',#10327);
#1901=VERTEX_POINT('',#10329);
#1902=VERTEX_POINT('',#10331);
#1903=VERTEX_POINT('',#10335);
#1904=VERTEX_POINT('',#10337);
#1905=VERTEX_POINT('',#10341);
#1906=VERTEX_POINT('',#10343);
#1907=VERTEX_POINT('',#10351);
#1908=VERTEX_POINT('',#10352);
#1909=VERTEX_POINT('',#10354);
#1910=VERTEX_POINT('',#10356);
#1911=VERTEX_POINT('',#10360);
#1912=VERTEX_POINT('',#10362);
#1913=VERTEX_POINT('',#10366);
#1914=VERTEX_POINT('',#10368);
#1915=VERTEX_POINT('',#10376);
#1916=VERTEX_POINT('',#10378);
#1917=VERTEX_POINT('',#10381);
#1918=VERTEX_POINT('',#10385);
#1919=VERTEX_POINT('',#10388);
#1920=VERTEX_POINT('',#10392);
#1921=VERTEX_POINT('',#10395);
#1922=VERTEX_POINT('',#10399);
#1923=VERTEX_POINT('',#10402);
#1924=VERTEX_POINT('',#10406);
#1925=VERTEX_POINT('',#10411);
#1926=VERTEX_POINT('',#10415);
#2251=EDGE_CURVE('',#1817,#1818,#1145,.T.);
#2252=EDGE_CURVE('',#1818,#1819,#1606,.T.);
#2253=EDGE_CURVE('',#1819,#1820,#960,.T.);
#2254=EDGE_CURVE('',#1820,#1817,#1607,.T.);
#2255=EDGE_CURVE('',#1821,#1822,#1146,.T.);
#2256=EDGE_CURVE('',#1822,#1818,#1608,.T.);
#2257=EDGE_CURVE('',#1817,#1821,#1609,.T.);
#2258=EDGE_CURVE('',#1823,#1824,#1147,.T.);
#2259=EDGE_CURVE('',#1824,#1822,#1610,.T.);
#2260=EDGE_CURVE('',#1821,#1823,#1611,.T.);
#2261=EDGE_CURVE('',#1825,#1826,#1148,.T.);
#2262=EDGE_CURVE('',#1826,#1824,#1612,.T.);
#2263=EDGE_CURVE('',#1823,#1825,#1613,.T.);
#2264=EDGE_CURVE('',#1827,#1828,#1149,.T.);
#2265=EDGE_CURVE('',#1828,#1826,#1614,.T.);
#2266=EDGE_CURVE('',#1825,#1827,#1615,.T.);
#2267=EDGE_CURVE('',#1829,#1830,#1150,.T.);
#2268=EDGE_CURVE('',#1830,#1828,#1616,.T.);
#2269=EDGE_CURVE('',#1827,#1829,#1617,.T.);
#2270=EDGE_CURVE('',#1831,#1832,#1151,.T.);
#2271=EDGE_CURVE('',#1832,#1830,#1618,.T.);
#2272=EDGE_CURVE('',#1829,#1831,#1619,.T.);
#2273=EDGE_CURVE('',#1833,#1834,#1152,.T.);
#2274=EDGE_CURVE('',#1834,#1832,#1620,.T.);
#2275=EDGE_CURVE('',#1831,#1833,#1621,.T.);
#2276=EDGE_CURVE('',#1835,#1836,#1153,.T.);
#2277=EDGE_CURVE('',#1836,#1834,#1622,.T.);
#2278=EDGE_CURVE('',#1833,#1835,#1623,.T.);
#2279=EDGE_CURVE('',#1837,#1838,#1154,.T.);
#2280=EDGE_CURVE('',#1838,#1836,#1624,.T.);
#2281=EDGE_CURVE('',#1835,#1837,#1625,.T.);
#2282=EDGE_CURVE('',#1839,#1840,#1155,.T.);
#2283=EDGE_CURVE('',#1840,#1838,#1626,.T.);
#2284=EDGE_CURVE('',#1837,#1839,#1627,.T.);
#2285=EDGE_CURVE('',#1841,#1842,#1156,.T.);
#2286=EDGE_CURVE('',#1842,#1840,#1628,.T.);
#2287=EDGE_CURVE('',#1839,#1841,#1629,.T.);
#2288=EDGE_CURVE('',#1843,#1844,#1157,.T.);
#2289=EDGE_CURVE('',#1844,#1842,#1630,.T.);
#2290=EDGE_CURVE('',#1841,#1843,#1631,.T.);
#2291=EDGE_CURVE('',#1845,#1846,#1158,.T.);
#2292=EDGE_CURVE('',#1846,#1844,#1632,.T.);
#2293=EDGE_CURVE('',#1843,#1845,#1633,.T.);
#2294=EDGE_CURVE('',#1847,#1848,#1159,.T.);
#2295=EDGE_CURVE('',#1848,#1846,#1634,.T.);
#2296=EDGE_CURVE('',#1845,#1847,#1635,.T.);
#2297=EDGE_CURVE('',#1849,#1850,#1160,.T.);
#2298=EDGE_CURVE('',#1850,#1848,#1636,.T.);
#2299=EDGE_CURVE('',#1847,#1849,#1637,.T.);
#2300=EDGE_CURVE('',#1851,#1852,#1161,.T.);
#2301=EDGE_CURVE('',#1851,#1853,#1638,.T.);
#2302=EDGE_CURVE('',#1854,#1853,#961,.T.);
#2303=EDGE_CURVE('',#1854,#1852,#1639,.T.);
#2304=EDGE_CURVE('',#1855,#1856,#1162,.T.);
#2305=EDGE_CURVE('',#1856,#1857,#1640,.T.);
#2306=EDGE_CURVE('',#1858,#1857,#962,.T.);
#2307=EDGE_CURVE('',#1855,#1858,#1641,.T.);
#2308=EDGE_CURVE('',#1859,#1860,#1163,.T.);
#2309=EDGE_CURVE('',#1860,#1856,#1642,.T.);
#2310=EDGE_CURVE('',#1859,#1855,#1643,.T.);
#2311=EDGE_CURVE('',#1861,#1862,#1164,.T.);
#2312=EDGE_CURVE('',#1862,#1860,#1644,.T.);
#2313=EDGE_CURVE('',#1861,#1859,#1645,.T.);
#2314=EDGE_CURVE('',#1863,#1864,#1165,.T.);
#2315=EDGE_CURVE('',#1864,#1862,#1646,.T.);
#2316=EDGE_CURVE('',#1863,#1861,#1647,.T.);
#2317=EDGE_CURVE('',#1865,#1866,#1166,.T.);
#2318=EDGE_CURVE('',#1866,#1864,#1648,.T.);
#2319=EDGE_CURVE('',#1865,#1863,#1649,.T.);
#2320=EDGE_CURVE('',#1867,#1868,#1167,.T.);
#2321=EDGE_CURVE('',#1868,#1866,#1650,.T.);
#2322=EDGE_CURVE('',#1867,#1865,#1651,.T.);
#2323=EDGE_CURVE('',#1869,#1870,#1168,.T.);
#2324=EDGE_CURVE('',#1870,#1868,#1652,.T.);
#2325=EDGE_CURVE('',#1869,#1867,#1653,.T.);
#2326=EDGE_CURVE('',#1871,#1872,#1169,.T.);
#2327=EDGE_CURVE('',#1872,#1870,#1654,.T.);
#2328=EDGE_CURVE('',#1871,#1869,#1655,.T.);
#2329=EDGE_CURVE('',#1873,#1874,#1170,.T.);
#2330=EDGE_CURVE('',#1874,#1872,#1656,.T.);
#2331=EDGE_CURVE('',#1873,#1871,#1657,.T.);
#2332=EDGE_CURVE('',#1875,#1876,#1171,.T.);
#2333=EDGE_CURVE('',#1876,#1874,#1658,.T.);
#2334=EDGE_CURVE('',#1875,#1873,#1659,.T.);
#2335=EDGE_CURVE('',#1877,#1878,#1172,.T.);
#2336=EDGE_CURVE('',#1878,#1876,#1660,.T.);
#2337=EDGE_CURVE('',#1877,#1875,#1661,.T.);
#2338=EDGE_CURVE('',#1879,#1880,#1173,.T.);
#2339=EDGE_CURVE('',#1880,#1878,#1662,.T.);
#2340=EDGE_CURVE('',#1879,#1877,#1663,.T.);
#2341=EDGE_CURVE('',#1881,#1882,#1174,.T.);
#2342=EDGE_CURVE('',#1882,#1880,#1664,.T.);
#2343=EDGE_CURVE('',#1881,#1879,#1665,.T.);
#2344=EDGE_CURVE('',#1883,#1884,#1175,.T.);
#2345=EDGE_CURVE('',#1884,#1882,#1666,.T.);
#2346=EDGE_CURVE('',#1883,#1881,#1667,.T.);
#2347=EDGE_CURVE('',#1885,#1886,#1176,.T.);
#2348=EDGE_CURVE('',#1886,#1884,#1668,.T.);
#2349=EDGE_CURVE('',#1885,#1883,#1669,.T.);
#2350=EDGE_CURVE('',#1887,#1888,#1177,.T.);
#2351=EDGE_CURVE('',#1888,#1886,#1670,.T.);
#2352=EDGE_CURVE('',#1887,#1885,#1671,.T.);
#2353=EDGE_CURVE('',#1889,#1890,#1178,.T.);
#2354=EDGE_CURVE('',#1890,#1888,#1672,.T.);
#2355=EDGE_CURVE('',#1889,#1887,#1673,.T.);
#2356=EDGE_CURVE('',#1891,#1892,#1179,.T.);
#2357=EDGE_CURVE('',#1893,#1891,#1674,.T.);
#2358=EDGE_CURVE('',#1894,#1893,#963,.T.);
#2359=EDGE_CURVE('',#1894,#1892,#1675,.T.);
#2360=EDGE_CURVE('',#1820,#1895,#964,.T.);
#2361=EDGE_CURVE('',#1895,#1819,#965,.T.);
#2362=EDGE_CURVE('',#1819,#1858,#1676,.T.);
#2363=EDGE_CURVE('',#1857,#1820,#1677,.T.);
#2364=EDGE_CURVE('',#1892,#1890,#1678,.T.);
#2365=EDGE_CURVE('',#1891,#1889,#1679,.T.);
#2366=EDGE_CURVE('',#1853,#1894,#1680,.T.);
#2367=EDGE_CURVE('',#1849,#1851,#1681,.T.);
#2368=EDGE_CURVE('',#1893,#1854,#1682,.T.);
#2369=EDGE_CURVE('',#1896,#1854,#966,.T.);
#2370=EDGE_CURVE('',#1853,#1896,#967,.T.);
#2371=EDGE_CURVE('',#1852,#1850,#1683,.T.);
#2372=EDGE_CURVE('',#1897,#1896,#1180,.T.);
#2373=EDGE_CURVE('',#1895,#1898,#1181,.T.);
#2374=EDGE_CURVE('',#1898,#1898,#968,.T.);
#2375=EDGE_CURVE('',#1899,#1900,#1182,.T.);
#2376=EDGE_CURVE('',#1901,#1899,#1183,.T.);
#2377=EDGE_CURVE('',#1902,#1901,#1184,.T.);
#2378=EDGE_CURVE('',#1900,#1902,#1185,.T.);
#2379=EDGE_CURVE('',#1900,#1903,#969,.T.);
#2380=EDGE_CURVE('',#1904,#1902,#1186,.T.);
#2381=EDGE_CURVE('',#1904,#1903,#1187,.T.);
#2382=EDGE_CURVE('',#1903,#1905,#1188,.T.);
#2383=EDGE_CURVE('',#1906,#1904,#1189,.T.);
#2384=EDGE_CURVE('',#1905,#1906,#1190,.T.);
#2385=EDGE_CURVE('',#1905,#1899,#970,.T.);
#2386=EDGE_CURVE('',#1906,#1901,#1191,.T.);
#2387=EDGE_CURVE('',#1907,#1908,#1192,.T.);
#2388=EDGE_CURVE('',#1909,#1907,#1193,.T.);
#2389=EDGE_CURVE('',#1910,#1909,#1194,.T.);
#2390=EDGE_CURVE('',#1908,#1910,#1195,.T.);
#2391=EDGE_CURVE('',#1908,#1911,#971,.T.);
#2392=EDGE_CURVE('',#1912,#1910,#1196,.T.);
#2393=EDGE_CURVE('',#1912,#1911,#1197,.T.);
#2394=EDGE_CURVE('',#1911,#1913,#1198,.T.);
#2395=EDGE_CURVE('',#1914,#1912,#1199,.T.);
#2396=EDGE_CURVE('',#1913,#1914,#1200,.T.);
#2397=EDGE_CURVE('',#1913,#1907,#972,.T.);
#2398=EDGE_CURVE('',#1914,#1909,#1201,.T.);
#2399=EDGE_CURVE('',#1915,#1915,#973,.T.);
#2400=EDGE_CURVE('',#1916,#1916,#974,.T.);
#2401=EDGE_CURVE('',#1917,#1917,#975,.T.);
#2402=EDGE_CURVE('',#1917,#1916,#1202,.T.);
#2403=EDGE_CURVE('',#1918,#1918,#976,.T.);
#2404=EDGE_CURVE('',#1918,#1919,#1203,.T.);
#2405=EDGE_CURVE('',#1919,#1919,#977,.T.);
#2406=EDGE_CURVE('',#1920,#1920,#978,.T.);
#2407=EDGE_CURVE('',#1921,#1921,#979,.T.);
#2408=EDGE_CURVE('',#1921,#1920,#1204,.T.);
#2409=EDGE_CURVE('',#1922,#1922,#980,.T.);
#2410=EDGE_CURVE('',#1922,#1923,#1205,.T.);
#2411=EDGE_CURVE('',#1923,#1923,#981,.T.);
#2412=EDGE_CURVE('',#1924,#1924,#982,.T.);
#2413=EDGE_CURVE('',#1923,#1924,#1206,.T.);
#2414=EDGE_CURVE('',#1925,#1925,#983,.T.);
#2415=EDGE_CURVE('',#1925,#1915,#1207,.T.);
#2416=EDGE_CURVE('',#1926,#1926,#984,.T.);
#2417=EDGE_CURVE('',#1926,#1925,#1208,.T.);
#2997=ORIENTED_EDGE('',*,*,#2251,.T.);
#2998=ORIENTED_EDGE('',*,*,#2252,.T.);
#2999=ORIENTED_EDGE('',*,*,#2253,.T.);
#3000=ORIENTED_EDGE('',*,*,#2254,.T.);
#3001=ORIENTED_EDGE('',*,*,#2255,.T.);
#3002=ORIENTED_EDGE('',*,*,#2256,.T.);
#3003=ORIENTED_EDGE('',*,*,#2251,.F.);
#3004=ORIENTED_EDGE('',*,*,#2257,.T.);
#3005=ORIENTED_EDGE('',*,*,#2258,.T.);
#3006=ORIENTED_EDGE('',*,*,#2259,.T.);
#3007=ORIENTED_EDGE('',*,*,#2255,.F.);
#3008=ORIENTED_EDGE('',*,*,#2260,.T.);
#3009=ORIENTED_EDGE('',*,*,#2261,.T.);
#3010=ORIENTED_EDGE('',*,*,#2262,.T.);
#3011=ORIENTED_EDGE('',*,*,#2258,.F.);
#3012=ORIENTED_EDGE('',*,*,#2263,.T.);
#3013=ORIENTED_EDGE('',*,*,#2264,.T.);
#3014=ORIENTED_EDGE('',*,*,#2265,.T.);
#3015=ORIENTED_EDGE('',*,*,#2261,.F.);
#3016=ORIENTED_EDGE('',*,*,#2266,.T.);
#3017=ORIENTED_EDGE('',*,*,#2267,.T.);
#3018=ORIENTED_EDGE('',*,*,#2268,.T.);
#3019=ORIENTED_EDGE('',*,*,#2264,.F.);
#3020=ORIENTED_EDGE('',*,*,#2269,.T.);
#3021=ORIENTED_EDGE('',*,*,#2270,.T.);
#3022=ORIENTED_EDGE('',*,*,#2271,.T.);
#3023=ORIENTED_EDGE('',*,*,#2267,.F.);
#3024=ORIENTED_EDGE('',*,*,#2272,.T.);
#3025=ORIENTED_EDGE('',*,*,#2273,.T.);
#3026=ORIENTED_EDGE('',*,*,#2274,.T.);
#3027=ORIENTED_EDGE('',*,*,#2270,.F.);
#3028=ORIENTED_EDGE('',*,*,#2275,.T.);
#3029=ORIENTED_EDGE('',*,*,#2276,.T.);
#3030=ORIENTED_EDGE('',*,*,#2277,.T.);
#3031=ORIENTED_EDGE('',*,*,#2273,.F.);
#3032=ORIENTED_EDGE('',*,*,#2278,.T.);
#3033=ORIENTED_EDGE('',*,*,#2279,.T.);
#3034=ORIENTED_EDGE('',*,*,#2280,.T.);
#3035=ORIENTED_EDGE('',*,*,#2276,.F.);
#3036=ORIENTED_EDGE('',*,*,#2281,.T.);
#3037=ORIENTED_EDGE('',*,*,#2282,.T.);
#3038=ORIENTED_EDGE('',*,*,#2283,.T.);
#3039=ORIENTED_EDGE('',*,*,#2279,.F.);
#3040=ORIENTED_EDGE('',*,*,#2284,.T.);
#3041=ORIENTED_EDGE('',*,*,#2285,.T.);
#3042=ORIENTED_EDGE('',*,*,#2286,.T.);
#3043=ORIENTED_EDGE('',*,*,#2282,.F.);
#3044=ORIENTED_EDGE('',*,*,#2287,.T.);
#3045=ORIENTED_EDGE('',*,*,#2288,.T.);
#3046=ORIENTED_EDGE('',*,*,#2289,.T.);
#3047=ORIENTED_EDGE('',*,*,#2285,.F.);
#3048=ORIENTED_EDGE('',*,*,#2290,.T.);
#3049=ORIENTED_EDGE('',*,*,#2291,.T.);
#3050=ORIENTED_EDGE('',*,*,#2292,.T.);
#3051=ORIENTED_EDGE('',*,*,#2288,.F.);
#3052=ORIENTED_EDGE('',*,*,#2293,.T.);
#3053=ORIENTED_EDGE('',*,*,#2294,.T.);
#3054=ORIENTED_EDGE('',*,*,#2295,.T.);
#3055=ORIENTED_EDGE('',*,*,#2291,.F.);
#3056=ORIENTED_EDGE('',*,*,#2296,.T.);
#3057=ORIENTED_EDGE('',*,*,#2297,.T.);
#3058=ORIENTED_EDGE('',*,*,#2298,.T.);
#3059=ORIENTED_EDGE('',*,*,#2294,.F.);
#3060=ORIENTED_EDGE('',*,*,#2299,.T.);
#3061=ORIENTED_EDGE('',*,*,#2300,.F.);
#3062=ORIENTED_EDGE('',*,*,#2301,.T.);
#3063=ORIENTED_EDGE('',*,*,#2302,.F.);
#3064=ORIENTED_EDGE('',*,*,#2303,.T.);
#3065=ORIENTED_EDGE('',*,*,#2304,.T.);
#3066=ORIENTED_EDGE('',*,*,#2305,.T.);
#3067=ORIENTED_EDGE('',*,*,#2306,.F.);
#3068=ORIENTED_EDGE('',*,*,#2307,.F.);
#3069=ORIENTED_EDGE('',*,*,#2308,.T.);
#3070=ORIENTED_EDGE('',*,*,#2309,.T.);
#3071=ORIENTED_EDGE('',*,*,#2304,.F.);
#3072=ORIENTED_EDGE('',*,*,#2310,.F.);
#3073=ORIENTED_EDGE('',*,*,#2311,.T.);
#3074=ORIENTED_EDGE('',*,*,#2312,.T.);
#3075=ORIENTED_EDGE('',*,*,#2308,.F.);
#3076=ORIENTED_EDGE('',*,*,#2313,.F.);
#3077=ORIENTED_EDGE('',*,*,#2314,.T.);
#3078=ORIENTED_EDGE('',*,*,#2315,.T.);
#3079=ORIENTED_EDGE('',*,*,#2311,.F.);
#3080=ORIENTED_EDGE('',*,*,#2316,.F.);
#3081=ORIENTED_EDGE('',*,*,#2317,.T.);
#3082=ORIENTED_EDGE('',*,*,#2318,.T.);
#3083=ORIENTED_EDGE('',*,*,#2314,.F.);
#3084=ORIENTED_EDGE('',*,*,#2319,.F.);
#3085=ORIENTED_EDGE('',*,*,#2320,.T.);
#3086=ORIENTED_EDGE('',*,*,#2321,.T.);
#3087=ORIENTED_EDGE('',*,*,#2317,.F.);
#3088=ORIENTED_EDGE('',*,*,#2322,.F.);
#3089=ORIENTED_EDGE('',*,*,#2323,.T.);
#3090=ORIENTED_EDGE('',*,*,#2324,.T.);
#3091=ORIENTED_EDGE('',*,*,#2320,.F.);
#3092=ORIENTED_EDGE('',*,*,#2325,.F.);
#3093=ORIENTED_EDGE('',*,*,#2326,.T.);
#3094=ORIENTED_EDGE('',*,*,#2327,.T.);
#3095=ORIENTED_EDGE('',*,*,#2323,.F.);
#3096=ORIENTED_EDGE('',*,*,#2328,.F.);
#3097=ORIENTED_EDGE('',*,*,#2329,.T.);
#3098=ORIENTED_EDGE('',*,*,#2330,.T.);
#3099=ORIENTED_EDGE('',*,*,#2326,.F.);
#3100=ORIENTED_EDGE('',*,*,#2331,.F.);
#3101=ORIENTED_EDGE('',*,*,#2332,.T.);
#3102=ORIENTED_EDGE('',*,*,#2333,.T.);
#3103=ORIENTED_EDGE('',*,*,#2329,.F.);
#3104=ORIENTED_EDGE('',*,*,#2334,.F.);
#3105=ORIENTED_EDGE('',*,*,#2335,.T.);
#3106=ORIENTED_EDGE('',*,*,#2336,.T.);
#3107=ORIENTED_EDGE('',*,*,#2332,.F.);
#3108=ORIENTED_EDGE('',*,*,#2337,.F.);
#3109=ORIENTED_EDGE('',*,*,#2338,.T.);
#3110=ORIENTED_EDGE('',*,*,#2339,.T.);
#3111=ORIENTED_EDGE('',*,*,#2335,.F.);
#3112=ORIENTED_EDGE('',*,*,#2340,.F.);
#3113=ORIENTED_EDGE('',*,*,#2341,.T.);
#3114=ORIENTED_EDGE('',*,*,#2342,.T.);
#3115=ORIENTED_EDGE('',*,*,#2338,.F.);
#3116=ORIENTED_EDGE('',*,*,#2343,.F.);
#3117=ORIENTED_EDGE('',*,*,#2344,.T.);
#3118=ORIENTED_EDGE('',*,*,#2345,.T.);
#3119=ORIENTED_EDGE('',*,*,#2341,.F.);
#3120=ORIENTED_EDGE('',*,*,#2346,.F.);
#3121=ORIENTED_EDGE('',*,*,#2347,.T.);
#3122=ORIENTED_EDGE('',*,*,#2348,.T.);
#3123=ORIENTED_EDGE('',*,*,#2344,.F.);
#3124=ORIENTED_EDGE('',*,*,#2349,.F.);
#3125=ORIENTED_EDGE('',*,*,#2350,.T.);
#3126=ORIENTED_EDGE('',*,*,#2351,.T.);
#3127=ORIENTED_EDGE('',*,*,#2347,.F.);
#3128=ORIENTED_EDGE('',*,*,#2352,.F.);
#3129=ORIENTED_EDGE('',*,*,#2353,.T.);
#3130=ORIENTED_EDGE('',*,*,#2354,.T.);
#3131=ORIENTED_EDGE('',*,*,#2350,.F.);
#3132=ORIENTED_EDGE('',*,*,#2355,.F.);
#3133=ORIENTED_EDGE('',*,*,#2356,.F.);
#3134=ORIENTED_EDGE('',*,*,#2357,.F.);
#3135=ORIENTED_EDGE('',*,*,#2358,.F.);
#3136=ORIENTED_EDGE('',*,*,#2359,.T.);
#3137=ORIENTED_EDGE('',*,*,#2360,.T.);
#3138=ORIENTED_EDGE('',*,*,#2361,.T.);
#3139=ORIENTED_EDGE('',*,*,#2362,.T.);
#3140=ORIENTED_EDGE('',*,*,#2306,.T.);
#3141=ORIENTED_EDGE('',*,*,#2363,.T.);
#3142=ORIENTED_EDGE('',*,*,#2356,.T.);
#3143=ORIENTED_EDGE('',*,*,#2364,.T.);
#3144=ORIENTED_EDGE('',*,*,#2353,.F.);
#3145=ORIENTED_EDGE('',*,*,#2365,.F.);
#3146=ORIENTED_EDGE('',*,*,#2363,.F.);
#3147=ORIENTED_EDGE('',*,*,#2305,.F.);
#3148=ORIENTED_EDGE('',*,*,#2309,.F.);
#3149=ORIENTED_EDGE('',*,*,#2312,.F.);
#3150=ORIENTED_EDGE('',*,*,#2315,.F.);
#3151=ORIENTED_EDGE('',*,*,#2318,.F.);
#3152=ORIENTED_EDGE('',*,*,#2321,.F.);
#3153=ORIENTED_EDGE('',*,*,#2324,.F.);
#3154=ORIENTED_EDGE('',*,*,#2327,.F.);
#3155=ORIENTED_EDGE('',*,*,#2330,.F.);
#3156=ORIENTED_EDGE('',*,*,#2333,.F.);
#3157=ORIENTED_EDGE('',*,*,#2336,.F.);
#3158=ORIENTED_EDGE('',*,*,#2339,.F.);
#3159=ORIENTED_EDGE('',*,*,#2342,.F.);
#3160=ORIENTED_EDGE('',*,*,#2345,.F.);
#3161=ORIENTED_EDGE('',*,*,#2348,.F.);
#3162=ORIENTED_EDGE('',*,*,#2351,.F.);
#3163=ORIENTED_EDGE('',*,*,#2354,.F.);
#3164=ORIENTED_EDGE('',*,*,#2364,.F.);
#3165=ORIENTED_EDGE('',*,*,#2359,.F.);
#3166=ORIENTED_EDGE('',*,*,#2366,.F.);
#3167=ORIENTED_EDGE('',*,*,#2301,.F.);
#3168=ORIENTED_EDGE('',*,*,#2367,.F.);
#3169=ORIENTED_EDGE('',*,*,#2299,.F.);
#3170=ORIENTED_EDGE('',*,*,#2296,.F.);
#3171=ORIENTED_EDGE('',*,*,#2293,.F.);
#3172=ORIENTED_EDGE('',*,*,#2290,.F.);
#3173=ORIENTED_EDGE('',*,*,#2287,.F.);
#3174=ORIENTED_EDGE('',*,*,#2284,.F.);
#3175=ORIENTED_EDGE('',*,*,#2281,.F.);
#3176=ORIENTED_EDGE('',*,*,#2278,.F.);
#3177=ORIENTED_EDGE('',*,*,#2275,.F.);
#3178=ORIENTED_EDGE('',*,*,#2272,.F.);
#3179=ORIENTED_EDGE('',*,*,#2269,.F.);
#3180=ORIENTED_EDGE('',*,*,#2266,.F.);
#3181=ORIENTED_EDGE('',*,*,#2263,.F.);
#3182=ORIENTED_EDGE('',*,*,#2260,.F.);
#3183=ORIENTED_EDGE('',*,*,#2257,.F.);
#3184=ORIENTED_EDGE('',*,*,#2254,.F.);
#3185=ORIENTED_EDGE('',*,*,#2358,.T.);
#3186=ORIENTED_EDGE('',*,*,#2368,.T.);
#3187=ORIENTED_EDGE('',*,*,#2369,.F.);
#3188=ORIENTED_EDGE('',*,*,#2370,.F.);
#3189=ORIENTED_EDGE('',*,*,#2366,.T.);
#3190=ORIENTED_EDGE('',*,*,#2362,.F.);
#3191=ORIENTED_EDGE('',*,*,#2252,.F.);
#3192=ORIENTED_EDGE('',*,*,#2256,.F.);
#3193=ORIENTED_EDGE('',*,*,#2259,.F.);
#3194=ORIENTED_EDGE('',*,*,#2262,.F.);
#3195=ORIENTED_EDGE('',*,*,#2265,.F.);
#3196=ORIENTED_EDGE('',*,*,#2268,.F.);
#3197=ORIENTED_EDGE('',*,*,#2271,.F.);
#3198=ORIENTED_EDGE('',*,*,#2274,.F.);
#3199=ORIENTED_EDGE('',*,*,#2277,.F.);
#3200=ORIENTED_EDGE('',*,*,#2280,.F.);
#3201=ORIENTED_EDGE('',*,*,#2283,.F.);
#3202=ORIENTED_EDGE('',*,*,#2286,.F.);
#3203=ORIENTED_EDGE('',*,*,#2289,.F.);
#3204=ORIENTED_EDGE('',*,*,#2292,.F.);
#3205=ORIENTED_EDGE('',*,*,#2295,.F.);
#3206=ORIENTED_EDGE('',*,*,#2298,.F.);
#3207=ORIENTED_EDGE('',*,*,#2371,.F.);
#3208=ORIENTED_EDGE('',*,*,#2303,.F.);
#3209=ORIENTED_EDGE('',*,*,#2368,.F.);
#3210=ORIENTED_EDGE('',*,*,#2357,.T.);
#3211=ORIENTED_EDGE('',*,*,#2365,.T.);
#3212=ORIENTED_EDGE('',*,*,#2355,.T.);
#3213=ORIENTED_EDGE('',*,*,#2352,.T.);
#3214=ORIENTED_EDGE('',*,*,#2349,.T.);
#3215=ORIENTED_EDGE('',*,*,#2346,.T.);
#3216=ORIENTED_EDGE('',*,*,#2343,.T.);
#3217=ORIENTED_EDGE('',*,*,#2340,.T.);
#3218=ORIENTED_EDGE('',*,*,#2337,.T.);
#3219=ORIENTED_EDGE('',*,*,#2334,.T.);
#3220=ORIENTED_EDGE('',*,*,#2331,.T.);
#3221=ORIENTED_EDGE('',*,*,#2328,.T.);
#3222=ORIENTED_EDGE('',*,*,#2325,.T.);
#3223=ORIENTED_EDGE('',*,*,#2322,.T.);
#3224=ORIENTED_EDGE('',*,*,#2319,.T.);
#3225=ORIENTED_EDGE('',*,*,#2316,.T.);
#3226=ORIENTED_EDGE('',*,*,#2313,.T.);
#3227=ORIENTED_EDGE('',*,*,#2310,.T.);
#3228=ORIENTED_EDGE('',*,*,#2307,.T.);
#3229=ORIENTED_EDGE('',*,*,#2372,.T.);
#3230=ORIENTED_EDGE('',*,*,#2369,.T.);
#3231=ORIENTED_EDGE('',*,*,#2302,.T.);
#3232=ORIENTED_EDGE('',*,*,#2370,.T.);
#3233=ORIENTED_EDGE('',*,*,#2372,.F.);
#3234=ORIENTED_EDGE('',*,*,#2300,.T.);
#3235=ORIENTED_EDGE('',*,*,#2371,.T.);
#3236=ORIENTED_EDGE('',*,*,#2297,.F.);
#3237=ORIENTED_EDGE('',*,*,#2367,.T.);
#3238=ORIENTED_EDGE('',*,*,#2360,.F.);
#3239=ORIENTED_EDGE('',*,*,#2253,.F.);
#3240=ORIENTED_EDGE('',*,*,#2361,.F.);
#3241=ORIENTED_EDGE('',*,*,#2373,.T.);
#3242=ORIENTED_EDGE('',*,*,#2374,.F.);
#3243=ORIENTED_EDGE('',*,*,#2373,.F.);
#3244=ORIENTED_EDGE('',*,*,#2375,.F.);
#3245=ORIENTED_EDGE('',*,*,#2376,.F.);
#3246=ORIENTED_EDGE('',*,*,#2377,.F.);
#3247=ORIENTED_EDGE('',*,*,#2378,.F.);
#3248=ORIENTED_EDGE('',*,*,#2379,.F.);
#3249=ORIENTED_EDGE('',*,*,#2378,.T.);
#3250=ORIENTED_EDGE('',*,*,#2380,.F.);
#3251=ORIENTED_EDGE('',*,*,#2381,.T.);
#3252=ORIENTED_EDGE('',*,*,#2382,.F.);
#3253=ORIENTED_EDGE('',*,*,#2381,.F.);
#3254=ORIENTED_EDGE('',*,*,#2383,.F.);
#3255=ORIENTED_EDGE('',*,*,#2384,.F.);
#3256=ORIENTED_EDGE('',*,*,#2385,.F.);
#3257=ORIENTED_EDGE('',*,*,#2384,.T.);
#3258=ORIENTED_EDGE('',*,*,#2386,.T.);
#3259=ORIENTED_EDGE('',*,*,#2376,.T.);
#3260=ORIENTED_EDGE('',*,*,#2386,.F.);
#3261=ORIENTED_EDGE('',*,*,#2383,.T.);
#3262=ORIENTED_EDGE('',*,*,#2380,.T.);
#3263=ORIENTED_EDGE('',*,*,#2377,.T.);
#3264=ORIENTED_EDGE('',*,*,#2387,.F.);
#3265=ORIENTED_EDGE('',*,*,#2388,.F.);
#3266=ORIENTED_EDGE('',*,*,#2389,.F.);
#3267=ORIENTED_EDGE('',*,*,#2390,.F.);
#3268=ORIENTED_EDGE('',*,*,#2391,.F.);
#3269=ORIENTED_EDGE('',*,*,#2390,.T.);
#3270=ORIENTED_EDGE('',*,*,#2392,.F.);
#3271=ORIENTED_EDGE('',*,*,#2393,.T.);
#3272=ORIENTED_EDGE('',*,*,#2394,.F.);
#3273=ORIENTED_EDGE('',*,*,#2393,.F.);
#3274=ORIENTED_EDGE('',*,*,#2395,.F.);
#3275=ORIENTED_EDGE('',*,*,#2396,.F.);
#3276=ORIENTED_EDGE('',*,*,#2397,.F.);
#3277=ORIENTED_EDGE('',*,*,#2396,.T.);
#3278=ORIENTED_EDGE('',*,*,#2398,.T.);
#3279=ORIENTED_EDGE('',*,*,#2388,.T.);
#3280=ORIENTED_EDGE('',*,*,#2398,.F.);
#3281=ORIENTED_EDGE('',*,*,#2395,.T.);
#3282=ORIENTED_EDGE('',*,*,#2392,.T.);
#3283=ORIENTED_EDGE('',*,*,#2389,.T.);
#3284=ORIENTED_EDGE('',*,*,#2399,.F.);
#3285=ORIENTED_EDGE('',*,*,#2400,.T.);
#3286=ORIENTED_EDGE('',*,*,#2401,.T.);
#3287=ORIENTED_EDGE('',*,*,#2402,.T.);
#3288=ORIENTED_EDGE('',*,*,#2400,.F.);
#3289=ORIENTED_EDGE('',*,*,#2402,.F.);
#3290=ORIENTED_EDGE('',*,*,#2403,.F.);
#3291=ORIENTED_EDGE('',*,*,#2401,.F.);
#3292=ORIENTED_EDGE('',*,*,#2403,.T.);
#3293=ORIENTED_EDGE('',*,*,#2404,.T.);
#3294=ORIENTED_EDGE('',*,*,#2405,.T.);
#3295=ORIENTED_EDGE('',*,*,#2404,.F.);
#3296=ORIENTED_EDGE('',*,*,#2382,.T.);
#3297=ORIENTED_EDGE('',*,*,#2385,.T.);
#3298=ORIENTED_EDGE('',*,*,#2375,.T.);
#3299=ORIENTED_EDGE('',*,*,#2379,.T.);
#3300=ORIENTED_EDGE('',*,*,#2394,.T.);
#3301=ORIENTED_EDGE('',*,*,#2397,.T.);
#3302=ORIENTED_EDGE('',*,*,#2387,.T.);
#3303=ORIENTED_EDGE('',*,*,#2391,.T.);
#3304=ORIENTED_EDGE('',*,*,#2405,.F.);
#3305=ORIENTED_EDGE('',*,*,#2406,.T.);
#3306=ORIENTED_EDGE('',*,*,#2407,.T.);
#3307=ORIENTED_EDGE('',*,*,#2408,.T.);
#3308=ORIENTED_EDGE('',*,*,#2406,.F.);
#3309=ORIENTED_EDGE('',*,*,#2408,.F.);
#3310=ORIENTED_EDGE('',*,*,#2409,.F.);
#3311=ORIENTED_EDGE('',*,*,#2407,.F.);
#3312=ORIENTED_EDGE('',*,*,#2409,.T.);
#3313=ORIENTED_EDGE('',*,*,#2410,.T.);
#3314=ORIENTED_EDGE('',*,*,#2411,.T.);
#3315=ORIENTED_EDGE('',*,*,#2410,.F.);
#3316=ORIENTED_EDGE('',*,*,#2412,.F.);
#3317=ORIENTED_EDGE('',*,*,#2411,.F.);
#3318=ORIENTED_EDGE('',*,*,#2413,.T.);
#3319=ORIENTED_EDGE('',*,*,#2412,.T.);
#3320=ORIENTED_EDGE('',*,*,#2413,.F.);
#3321=ORIENTED_EDGE('',*,*,#2414,.F.);
#3322=ORIENTED_EDGE('',*,*,#2415,.T.);
#3323=ORIENTED_EDGE('',*,*,#2399,.T.);
#3324=ORIENTED_EDGE('',*,*,#2415,.F.);
#3325=ORIENTED_EDGE('',*,*,#2416,.F.);
#3326=ORIENTED_EDGE('',*,*,#2417,.T.);
#3327=ORIENTED_EDGE('',*,*,#2414,.T.);
#3328=ORIENTED_EDGE('',*,*,#2417,.F.);
#3329=ORIENTED_EDGE('',*,*,#2416,.T.);
#3330=ORIENTED_EDGE('',*,*,#2374,.T.);
#4040=CYLINDRICAL_SURFACE('',#4615,3.4544);
#4041=CYLINDRICAL_SURFACE('',#4617,3.4544);
#4042=CYLINDRICAL_SURFACE('',#4618,3.4544);
#4043=CYLINDRICAL_SURFACE('',#4619,3.4544);
#4044=CYLINDRICAL_SURFACE('',#4620,3.4544);
#4045=CYLINDRICAL_SURFACE('',#4621,3.4544);
#4046=CYLINDRICAL_SURFACE('',#4622,3.4544);
#4047=CYLINDRICAL_SURFACE('',#4623,3.4544);
#4048=CYLINDRICAL_SURFACE('',#4624,3.4544);
#4049=CYLINDRICAL_SURFACE('',#4625,3.4544);
#4050=CYLINDRICAL_SURFACE('',#4626,3.4544);
#4051=CYLINDRICAL_SURFACE('',#4627,3.4544);
#4052=CYLINDRICAL_SURFACE('',#4628,3.4544);
#4053=CYLINDRICAL_SURFACE('',#4629,3.4544);
#4054=CYLINDRICAL_SURFACE('',#4630,3.4544);
#4055=CYLINDRICAL_SURFACE('',#4631,3.4544);
#4056=CYLINDRICAL_SURFACE('',#4632,3.4544);
#4057=CYLINDRICAL_SURFACE('',#4634,3.96875);
#4058=CYLINDRICAL_SURFACE('',#4636,3.96875);
#4059=CYLINDRICAL_SURFACE('',#4637,3.96875);
#4060=CYLINDRICAL_SURFACE('',#4638,3.96875);
#4061=CYLINDRICAL_SURFACE('',#4639,3.96875);
#4062=CYLINDRICAL_SURFACE('',#4640,3.96875);
#4063=CYLINDRICAL_SURFACE('',#4641,3.96875);
#4064=CYLINDRICAL_SURFACE('',#4642,3.96875);
#4065=CYLINDRICAL_SURFACE('',#4643,3.96875);
#4066=CYLINDRICAL_SURFACE('',#4644,3.96875);
#4067=CYLINDRICAL_SURFACE('',#4645,3.96875);
#4068=CYLINDRICAL_SURFACE('',#4646,3.96875);
#4069=CYLINDRICAL_SURFACE('',#4647,3.96875);
#4070=CYLINDRICAL_SURFACE('',#4648,3.96875);
#4071=CYLINDRICAL_SURFACE('',#4649,3.96875);
#4072=CYLINDRICAL_SURFACE('',#4650,3.96875);
#4073=CYLINDRICAL_SURFACE('',#4651,3.96875);
#4074=CYLINDRICAL_SURFACE('',#4652,3.96875);
#4075=CYLINDRICAL_SURFACE('',#4657,3.96875);
#4076=CYLINDRICAL_SURFACE('',#4662,3.4544);
#4077=CYLINDRICAL_SURFACE('',#4682,7.6);
#4078=CYLINDRICAL_SURFACE('',#4686,7.94);
#4079=CYLINDRICAL_SURFACE('',#4690,7.6);
#4080=CYLINDRICAL_SURFACE('',#4694,7.94);
#4081=CYLINDRICAL_SURFACE('',#4699,7.94);
#4162=ADVANCED_FACE('',(#372),#4040,.F.);
#4163=ADVANCED_FACE('',(#373),#4041,.F.);
#4164=ADVANCED_FACE('',(#374),#4042,.F.);
#4165=ADVANCED_FACE('',(#375),#4043,.F.);
#4166=ADVANCED_FACE('',(#376),#4044,.F.);
#4167=ADVANCED_FACE('',(#377),#4045,.F.);
#4168=ADVANCED_FACE('',(#378),#4046,.F.);
#4169=ADVANCED_FACE('',(#379),#4047,.F.);
#4170=ADVANCED_FACE('',(#380),#4048,.F.);
#4171=ADVANCED_FACE('',(#381),#4049,.F.);
#4172=ADVANCED_FACE('',(#382),#4050,.F.);
#4173=ADVANCED_FACE('',(#383),#4051,.F.);
#4174=ADVANCED_FACE('',(#384),#4052,.F.);
#4175=ADVANCED_FACE('',(#385),#4053,.F.);
#4176=ADVANCED_FACE('',(#386),#4054,.F.);
#4177=ADVANCED_FACE('',(#387),#4055,.F.);
#4178=ADVANCED_FACE('',(#388),#4056,.F.);
#4179=ADVANCED_FACE('',(#389),#4057,.F.);
#4180=ADVANCED_FACE('',(#390),#4058,.F.);
#4181=ADVANCED_FACE('',(#391),#4059,.F.);
#4182=ADVANCED_FACE('',(#392),#4060,.F.);
#4183=ADVANCED_FACE('',(#393),#4061,.F.);
#4184=ADVANCED_FACE('',(#394),#4062,.F.);
#4185=ADVANCED_FACE('',(#395),#4063,.F.);
#4186=ADVANCED_FACE('',(#396),#4064,.F.);
#4187=ADVANCED_FACE('',(#397),#4065,.F.);
#4188=ADVANCED_FACE('',(#398),#4066,.F.);
#4189=ADVANCED_FACE('',(#399),#4067,.F.);
#4190=ADVANCED_FACE('',(#400),#4068,.F.);
#4191=ADVANCED_FACE('',(#401),#4069,.F.);
#4192=ADVANCED_FACE('',(#402),#4070,.F.);
#4193=ADVANCED_FACE('',(#403),#4071,.F.);
#4194=ADVANCED_FACE('',(#404),#4072,.F.);
#4195=ADVANCED_FACE('',(#405),#4073,.F.);
#4196=ADVANCED_FACE('',(#406),#4074,.F.);
#4197=ADVANCED_FACE('',(#407),#178,.F.);
#4198=ADVANCED_FACE('',(#408),#4075,.F.);
#4199=ADVANCED_FACE('',(#409),#306,.F.);
#4200=ADVANCED_FACE('',(#410),#179,.T.);
#4201=ADVANCED_FACE('',(#411),#307,.F.);
#4202=ADVANCED_FACE('',(#412),#85,.F.);
#4203=ADVANCED_FACE('',(#413),#4076,.F.);
#4204=ADVANCED_FACE('',(#414),#86,.F.);
#4205=ADVANCED_FACE('',(#415),#180,.F.);
#4206=ADVANCED_FACE('',(#416),#181,.F.);
#4207=ADVANCED_FACE('',(#417),#182,.F.);
#4208=ADVANCED_FACE('',(#418),#183,.F.);
#4209=ADVANCED_FACE('',(#419),#184,.F.);
#4210=ADVANCED_FACE('',(#420),#185,.F.);
#4211=ADVANCED_FACE('',(#421),#186,.F.);
#4212=ADVANCED_FACE('',(#422),#187,.F.);
#4213=ADVANCED_FACE('',(#423),#188,.F.);
#4214=ADVANCED_FACE('',(#424),#189,.F.);
#4215=ADVANCED_FACE('',(#425,#146),#190,.F.);
#4216=ADVANCED_FACE('',(#426),#4077,.T.);
#4217=ADVANCED_FACE('',(#427,#147),#191,.F.);
#4218=ADVANCED_FACE('',(#428,#148,#149),#4078,.T.);
#4219=ADVANCED_FACE('',(#429,#150),#192,.F.);
#4220=ADVANCED_FACE('',(#430),#4079,.T.);
#4221=ADVANCED_FACE('',(#431,#151),#193,.F.);
#4222=ADVANCED_FACE('',(#432),#4080,.T.);
#4223=ADVANCED_FACE('',(#433),#194,.T.);
#4224=ADVANCED_FACE('',(#434),#87,.T.);
#4225=ADVANCED_FACE('',(#435),#4081,.T.);
#4226=ADVANCED_FACE('',(#436),#88,.T.);
#4227=ADVANCED_FACE('',(#437,#152),#195,.T.);
#4386=CLOSED_SHELL('',(#4162,#4163,#4164,#4165,#4166,#4167,#4168,#4169,
#4170,#4171,#4172,#4173,#4174,#4175,#4176,#4177,#4178,#4179,#4180,#4181,
#4182,#4183,#4184,#4185,#4186,#4187,#4188,#4189,#4190,#4191,#4192,#4193,
#4194,#4195,#4196,#4197,#4198,#4199,#4200,#4201,#4202,#4203,#4204,#4205,
#4206,#4207,#4208,#4209,#4210,#4211,#4212,#4213,#4214,#4215,#4216,#4217,
#4218,#4219,#4220,#4221,#4222,#4223,#4224,#4225,#4226,#4227));
#4614=AXIS2_PLACEMENT_3D('',#7731,#5244,#5245);
#4615=AXIS2_PLACEMENT_3D('',#7732,#5246,#5247);
#4616=AXIS2_PLACEMENT_3D('',#7751,#5249,#5250);
#4617=AXIS2_PLACEMENT_3D('',#7774,#5251,#5252);
#4618=AXIS2_PLACEMENT_3D('',#7822,#5254,#5255);
#4619=AXIS2_PLACEMENT_3D('',#7873,#5257,#5258);
#4620=AXIS2_PLACEMENT_3D('',#7924,#5260,#5261);
#4621=AXIS2_PLACEMENT_3D('',#7972,#5263,#5264);
#4622=AXIS2_PLACEMENT_3D('',#8023,#5266,#5267);
#4623=AXIS2_PLACEMENT_3D('',#8071,#5269,#5270);
#4624=AXIS2_PLACEMENT_3D('',#8122,#5272,#5273);
#4625=AXIS2_PLACEMENT_3D('',#8173,#5275,#5276);
#4626=AXIS2_PLACEMENT_3D('',#8221,#5278,#5279);
#4627=AXIS2_PLACEMENT_3D('',#8272,#5281,#5282);
#4628=AXIS2_PLACEMENT_3D('',#8323,#5284,#5285);
#4629=AXIS2_PLACEMENT_3D('',#8371,#5287,#5288);
#4630=AXIS2_PLACEMENT_3D('',#8422,#5290,#5291);
#4631=AXIS2_PLACEMENT_3D('',#8470,#5293,#5294);
#4632=AXIS2_PLACEMENT_3D('',#8521,#5296,#5297);
#4633=AXIS2_PLACEMENT_3D('',#8540,#5299,#5300);
#4634=AXIS2_PLACEMENT_3D('',#8563,#5301,#5302);
#4635=AXIS2_PLACEMENT_3D('',#8573,#5304,#5305);
#4636=AXIS2_PLACEMENT_3D('',#8580,#5306,#5307);
#4637=AXIS2_PLACEMENT_3D('',#8605,#5309,#5310);
#4638=AXIS2_PLACEMENT_3D('',#8630,#5312,#5313);
#4639=AXIS2_PLACEMENT_3D('',#8654,#5315,#5316);
#4640=AXIS2_PLACEMENT_3D('',#8679,#5318,#5319);
#4641=AXIS2_PLACEMENT_3D('',#8704,#5321,#5322);
#4642=AXIS2_PLACEMENT_3D('',#8728,#5324,#5325);
#4643=AXIS2_PLACEMENT_3D('',#8752,#5327,#5328);
#4644=AXIS2_PLACEMENT_3D('',#8778,#5330,#5331);
#4645=AXIS2_PLACEMENT_3D('',#8802,#5333,#5334);
#4646=AXIS2_PLACEMENT_3D('',#8826,#5336,#5337);
#4647=AXIS2_PLACEMENT_3D('',#8852,#5339,#5340);
#4648=AXIS2_PLACEMENT_3D('',#8876,#5342,#5343);
#4649=AXIS2_PLACEMENT_3D('',#8900,#5345,#5346);
#4650=AXIS2_PLACEMENT_3D('',#8925,#5348,#5349);
#4651=AXIS2_PLACEMENT_3D('',#8950,#5351,#5352);
#4652=AXIS2_PLACEMENT_3D('',#8974,#5354,#5355);
#4653=AXIS2_PLACEMENT_3D('',#8985,#5357,#5358);
#4654=AXIS2_PLACEMENT_3D('',#8992,#5359,#5360);
#4655=AXIS2_PLACEMENT_3D('',#8994,#5361,#5362);
#4656=AXIS2_PLACEMENT_3D('',#8995,#5363,#5364);
#4657=AXIS2_PLACEMENT_3D('',#9160,#5365,#5366);
#4658=AXIS2_PLACEMENT_3D('',#9749,#5367,#5368);
#4659=AXIS2_PLACEMENT_3D('',#9833,#5369,#5370);
#4660=AXIS2_PLACEMENT_3D('',#9834,#5371,#5372);
#4661=AXIS2_PLACEMENT_3D('',#10317,#5373,#5374);
#4662=AXIS2_PLACEMENT_3D('',#10320,#5376,#5377);
#4663=AXIS2_PLACEMENT_3D('',#10321,#5378,#5379);
#4664=AXIS2_PLACEMENT_3D('',#10324,#5381,#5382);
#4665=AXIS2_PLACEMENT_3D('',#10325,#5383,#5384);
#4666=AXIS2_PLACEMENT_3D('',#10334,#5389,#5390);
#4667=AXIS2_PLACEMENT_3D('',#10336,#5391,#5392);
#4668=AXIS2_PLACEMENT_3D('',#10340,#5395,#5396);
#4669=AXIS2_PLACEMENT_3D('',#10346,#5400,#5401);
#4670=AXIS2_PLACEMENT_3D('',#10347,#5402,#5403);
#4671=AXIS2_PLACEMENT_3D('',#10349,#5405,#5406);
#4672=AXIS2_PLACEMENT_3D('',#10350,#5407,#5408);
#4673=AXIS2_PLACEMENT_3D('',#10359,#5413,#5414);
#4674=AXIS2_PLACEMENT_3D('',#10361,#5415,#5416);
#4675=AXIS2_PLACEMENT_3D('',#10365,#5419,#5420);
#4676=AXIS2_PLACEMENT_3D('',#10371,#5424,#5425);
#4677=AXIS2_PLACEMENT_3D('',#10372,#5426,#5427);
#4678=AXIS2_PLACEMENT_3D('',#10374,#5429,#5430);
#4679=AXIS2_PLACEMENT_3D('',#10375,#5431,#5432);
#4680=AXIS2_PLACEMENT_3D('',#10377,#5433,#5434);
#4681=AXIS2_PLACEMENT_3D('',#10379,#5435,#5436);
#4682=AXIS2_PLACEMENT_3D('',#10380,#5437,#5438);
#4683=AXIS2_PLACEMENT_3D('',#10382,#5439,#5440);
#4684=AXIS2_PLACEMENT_3D('',#10384,#5442,#5443);
#4685=AXIS2_PLACEMENT_3D('',#10386,#5444,#5445);
#4686=AXIS2_PLACEMENT_3D('',#10387,#5446,#5447);
#4687=AXIS2_PLACEMENT_3D('',#10390,#5449,#5450);
#4688=AXIS2_PLACEMENT_3D('',#10391,#5451,#5452);
#4689=AXIS2_PLACEMENT_3D('',#10393,#5453,#5454);
#4690=AXIS2_PLACEMENT_3D('',#10394,#5455,#5456);
#4691=AXIS2_PLACEMENT_3D('',#10396,#5457,#5458);
#4692=AXIS2_PLACEMENT_3D('',#10398,#5460,#5461);
#4693=AXIS2_PLACEMENT_3D('',#10400,#5462,#5463);
#4694=AXIS2_PLACEMENT_3D('',#10401,#5464,#5465);
#4695=AXIS2_PLACEMENT_3D('',#10404,#5467,#5468);
#4696=AXIS2_PLACEMENT_3D('',#10405,#5469,#5470);
#4697=AXIS2_PLACEMENT_3D('',#10407,#5471,#5472);
#4698=AXIS2_PLACEMENT_3D('',#10408,#5473,#5474);
#4699=AXIS2_PLACEMENT_3D('',#10410,#5476,#5477);
#4700=AXIS2_PLACEMENT_3D('',#10412,#5478,#5479);
#4701=AXIS2_PLACEMENT_3D('',#10414,#5481,#5482);
#4702=AXIS2_PLACEMENT_3D('',#10416,#5483,#5484);
#4703=AXIS2_PLACEMENT_3D('',#10418,#5486,#5487);
#5244=DIRECTION('axis',(0.,0.,1.));
#5245=DIRECTION('refdir',(1.,0.,0.));
#5246=DIRECTION('center_axis',(1.,0.,0.));
#5247=DIRECTION('ref_axis',(0.,0.86829599907613,-0.496046427250903));
#5248=DIRECTION('',(1.,0.,0.));
#5249=DIRECTION('center_axis',(1.,0.,0.));
#5250=DIRECTION('ref_axis',(0.,1.,0.));
#5251=DIRECTION('center_axis',(1.,0.,0.));
#5252=DIRECTION('ref_axis',(0.,1.,0.));
#5253=DIRECTION('',(1.,0.,0.));
#5254=DIRECTION('center_axis',(1.,0.,0.));
#5255=DIRECTION('ref_axis',(0.,1.,0.));
#5256=DIRECTION('',(1.,0.,0.));
#5257=DIRECTION('center_axis',(1.,0.,0.));
#5258=DIRECTION('ref_axis',(0.,1.,0.));
#5259=DIRECTION('',(1.,0.,0.));
#5260=DIRECTION('center_axis',(1.,0.,0.));
#5261=DIRECTION('ref_axis',(0.,1.,0.));
#5262=DIRECTION('',(1.,0.,0.));
#5263=DIRECTION('center_axis',(1.,0.,0.));
#5264=DIRECTION('ref_axis',(0.,1.,0.));
#5265=DIRECTION('',(1.,0.,0.));
#5266=DIRECTION('center_axis',(1.,0.,0.));
#5267=DIRECTION('ref_axis',(0.,1.,0.));
#5268=DIRECTION('',(1.,0.,0.));
#5269=DIRECTION('center_axis',(1.,0.,0.));
#5270=DIRECTION('ref_axis',(0.,1.,0.));
#5271=DIRECTION('',(1.,0.,0.));
#5272=DIRECTION('center_axis',(1.,0.,0.));
#5273=DIRECTION('ref_axis',(0.,1.,0.));
#5274=DIRECTION('',(1.,0.,0.));
#5275=DIRECTION('center_axis',(1.,0.,0.));
#5276=DIRECTION('ref_axis',(0.,1.,0.));
#5277=DIRECTION('',(1.,0.,0.));
#5278=DIRECTION('center_axis',(1.,0.,0.));
#5279=DIRECTION('ref_axis',(0.,1.,0.));
#5280=DIRECTION('',(1.,0.,0.));
#5281=DIRECTION('center_axis',(1.,0.,0.));
#5282=DIRECTION('ref_axis',(0.,1.,0.));
#5283=DIRECTION('',(1.,0.,0.));
#5284=DIRECTION('center_axis',(1.,0.,0.));
#5285=DIRECTION('ref_axis',(0.,1.,0.));
#5286=DIRECTION('',(1.,0.,0.));
#5287=DIRECTION('center_axis',(1.,0.,0.));
#5288=DIRECTION('ref_axis',(0.,1.,0.));
#5289=DIRECTION('',(1.,0.,0.));
#5290=DIRECTION('center_axis',(1.,0.,0.));
#5291=DIRECTION('ref_axis',(0.,1.,0.));
#5292=DIRECTION('',(1.,0.,0.));
#5293=DIRECTION('center_axis',(1.,0.,0.));
#5294=DIRECTION('ref_axis',(0.,1.,0.));
#5295=DIRECTION('',(1.,0.,0.));
#5296=DIRECTION('center_axis',(1.,0.,0.));
#5297=DIRECTION('ref_axis',(0.,0.941324933064923,0.337501659833428));
#5298=DIRECTION('',(1.,0.,0.));
#5299=DIRECTION('center_axis',(1.,0.,0.));
#5300=DIRECTION('ref_axis',(0.,1.,0.));
#5301=DIRECTION('center_axis',(1.,0.,0.));
#5302=DIRECTION('ref_axis',(0.,-0.654392380830797,-0.75615515068708));
#5303=DIRECTION('',(1.,1.22464679914735E-16,1.26773667528936E-29));
#5304=DIRECTION('center_axis',(-1.,0.,0.));
#5305=DIRECTION('ref_axis',(0.,1.,1.03396090724959E-13));
#5306=DIRECTION('center_axis',(1.,0.,0.));
#5307=DIRECTION('ref_axis',(0.,1.,1.03396090724959E-13));
#5308=DIRECTION('',(1.,1.22464679914735E-16,1.26773667528936E-29));
#5309=DIRECTION('center_axis',(1.,0.,0.));
#5310=DIRECTION('ref_axis',(0.,1.,1.03396090724959E-13));
#5311=DIRECTION('',(1.,1.22464679914735E-16,1.26773667528936E-29));
#5312=DIRECTION('center_axis',(1.,0.,0.));
#5313=DIRECTION('ref_axis',(0.,1.,1.03396090724959E-13));
#5314=DIRECTION('',(1.,1.22464679914735E-16,1.26773667528936E-29));
#5315=DIRECTION('center_axis',(1.,0.,0.));
#5316=DIRECTION('ref_axis',(0.,1.,1.03396090724959E-13));
#5317=DIRECTION('',(1.,1.22464679914735E-16,1.26773667528936E-29));
#5318=DIRECTION('center_axis',(1.,0.,0.));
#5319=DIRECTION('ref_axis',(0.,1.,1.03396090724959E-13));
#5320=DIRECTION('',(1.,1.22464679914735E-16,1.26773667528936E-29));
#5321=DIRECTION('center_axis',(1.,0.,0.));
#5322=DIRECTION('ref_axis',(0.,1.,1.03396090724959E-13));
#5323=DIRECTION('',(1.,1.22464679914735E-16,1.26773667528936E-29));
#5324=DIRECTION('center_axis',(1.,0.,0.));
#5325=DIRECTION('ref_axis',(0.,1.,1.03396090724959E-13));
#5326=DIRECTION('',(1.,1.22464679914735E-16,1.26773667528936E-29));
#5327=DIRECTION('center_axis',(1.,0.,0.));
#5328=DIRECTION('ref_axis',(0.,1.,1.03396090724959E-13));
#5329=DIRECTION('',(1.,1.22464679914735E-16,1.26773667528936E-29));
#5330=DIRECTION('center_axis',(1.,0.,0.));
#5331=DIRECTION('ref_axis',(0.,1.,1.03396090724959E-13));
#5332=DIRECTION('',(1.,1.22464679914735E-16,1.26773667528936E-29));
#5333=DIRECTION('center_axis',(1.,0.,0.));
#5334=DIRECTION('ref_axis',(0.,1.,1.03396090724959E-13));
#5335=DIRECTION('',(1.,1.22464679914735E-16,1.26773667528936E-29));
#5336=DIRECTION('center_axis',(1.,0.,0.));
#5337=DIRECTION('ref_axis',(0.,1.,1.03396090724959E-13));
#5338=DIRECTION('',(1.,1.22464679914735E-16,1.26773667528936E-29));
#5339=DIRECTION('center_axis',(1.,0.,0.));
#5340=DIRECTION('ref_axis',(0.,1.,1.03396090724959E-13));
#5341=DIRECTION('',(1.,1.22464679914735E-16,1.26773667528936E-29));
#5342=DIRECTION('center_axis',(1.,0.,0.));
#5343=DIRECTION('ref_axis',(0.,1.,1.03396090724959E-13));
#5344=DIRECTION('',(1.,1.22464679914735E-16,1.26773667528936E-29));
#5345=DIRECTION('center_axis',(1.,0.,0.));
#5346=DIRECTION('ref_axis',(0.,1.,1.03396090724959E-13));
#5347=DIRECTION('',(1.,1.22464679914735E-16,1.26773667528936E-29));
#5348=DIRECTION('center_axis',(1.,0.,0.));
#5349=DIRECTION('ref_axis',(0.,1.,1.03396090724959E-13));
#5350=DIRECTION('',(1.,1.22464679914735E-16,1.26773667528936E-29));
#5351=DIRECTION('center_axis',(1.,0.,0.));
#5352=DIRECTION('ref_axis',(0.,1.,1.03396090724959E-13));
#5353=DIRECTION('',(1.,1.22464679914735E-16,1.26773667528936E-29));
#5354=DIRECTION('center_axis',(1.,0.,0.));
#5355=DIRECTION('ref_axis',(0.,-0.512398366081367,0.85874787594331));
#5356=DIRECTION('',(1.,1.22464679914735E-16,1.26773667528936E-29));
#5357=DIRECTION('center_axis',(1.,0.,0.));
#5358=DIRECTION('ref_axis',(0.,1.,1.03396090724959E-13));
#5359=DIRECTION('center_axis',(1.,0.,0.));
#5360=DIRECTION('ref_axis',(0.,0.,-1.));
#5361=DIRECTION('center_axis',(1.,0.,0.));
#5362=DIRECTION('ref_axis',(0.,1.,0.));
#5363=DIRECTION('center_axis',(1.,0.,0.));
#5364=DIRECTION('ref_axis',(0.,1.,0.));
#5365=DIRECTION('center_axis',(1.,0.,0.));
#5366=DIRECTION('ref_axis',(0.,1.,1.03396090724959E-13));
#5367=DIRECTION('center_axis',(1.,0.,0.));
#5368=DIRECTION('ref_axis',(0.,0.,-1.));
#5369=DIRECTION('center_axis',(1.,0.,0.));
#5370=DIRECTION('ref_axis',(0.,1.,0.));
#5371=DIRECTION('center_axis',(1.,0.,0.));
#5372=DIRECTION('ref_axis',(0.,1.,0.));
#5373=DIRECTION('center_axis',(1.,0.,0.));
#5374=DIRECTION('ref_axis',(0.,1.,0.));
#5375=DIRECTION('',(0.515038074910053,-0.857167300702113,-1.04972719113862E-16));
#5376=DIRECTION('center_axis',(1.,0.,0.));
#5377=DIRECTION('ref_axis',(0.,1.,0.));
#5378=DIRECTION('center_axis',(1.,0.,0.));
#5379=DIRECTION('ref_axis',(0.,1.,0.));
#5380=DIRECTION('',(0.70710678118654,-0.707106781186555,-8.65956056235502E-17));
#5381=DIRECTION('center_axis',(-1.,0.,0.));
#5382=DIRECTION('ref_axis',(0.,1.,0.));
#5383=DIRECTION('center_axis',(0.,0.,1.));
#5384=DIRECTION('ref_axis',(1.,0.,0.));
#5385=DIRECTION('',(-1.,0.,0.));
#5386=DIRECTION('',(0.,1.,0.));
#5387=DIRECTION('',(1.,0.,0.));
#5388=DIRECTION('',(0.,-1.,0.));
#5389=DIRECTION('center_axis',(-1.,0.,0.));
#5390=DIRECTION('ref_axis',(0.,-1.,0.));
#5391=DIRECTION('center_axis',(-1.,0.,0.));
#5392=DIRECTION('ref_axis',(0.,1.,0.));
#5393=DIRECTION('',(0.,0.,1.));
#5394=DIRECTION('',(0.,1.,0.));
#5395=DIRECTION('center_axis',(0.,0.,-1.));
#5396=DIRECTION('ref_axis',(-1.,0.,0.));
#5397=DIRECTION('',(1.,0.,0.));
#5398=DIRECTION('',(-1.,0.,0.));
#5399=DIRECTION('',(0.,-1.,0.));
#5400=DIRECTION('center_axis',(1.,0.,0.));
#5401=DIRECTION('ref_axis',(0.,1.,0.));
#5402=DIRECTION('center_axis',(1.,0.,0.));
#5403=DIRECTION('ref_axis',(0.,1.,0.));
#5404=DIRECTION('',(0.,0.,1.));
#5405=DIRECTION('center_axis',(0.,-1.,0.));
#5406=DIRECTION('ref_axis',(1.,0.,0.));
#5407=DIRECTION('center_axis',(0.,0.,1.));
#5408=DIRECTION('ref_axis',(1.,0.,0.));
#5409=DIRECTION('',(-1.,0.,0.));
#5410=DIRECTION('',(0.,1.,0.));
#5411=DIRECTION('',(1.,0.,0.));
#5412=DIRECTION('',(0.,-1.,0.));
#5413=DIRECTION('center_axis',(-1.,0.,0.));
#5414=DIRECTION('ref_axis',(0.,-1.,0.));
#5415=DIRECTION('center_axis',(-1.,0.,0.));
#5416=DIRECTION('ref_axis',(0.,1.,0.));
#5417=DIRECTION('',(0.,0.,1.));
#5418=DIRECTION('',(0.,1.,0.));
#5419=DIRECTION('center_axis',(0.,0.,-1.));
#5420=DIRECTION('ref_axis',(-1.,0.,0.));
#5421=DIRECTION('',(1.,0.,0.));
#5422=DIRECTION('',(-1.,0.,0.));
#5423=DIRECTION('',(0.,-1.,0.));
#5424=DIRECTION('center_axis',(1.,0.,0.));
#5425=DIRECTION('ref_axis',(0.,1.,0.));
#5426=DIRECTION('center_axis',(1.,0.,0.));
#5427=DIRECTION('ref_axis',(0.,1.,0.));
#5428=DIRECTION('',(0.,0.,1.));
#5429=DIRECTION('center_axis',(0.,-1.,0.));
#5430=DIRECTION('ref_axis',(1.,0.,0.));
#5431=DIRECTION('center_axis',(1.,0.,0.));
#5432=DIRECTION('ref_axis',(0.,0.,-1.));
#5433=DIRECTION('center_axis',(1.,0.,0.));
#5434=DIRECTION('ref_axis',(0.,1.,0.));
#5435=DIRECTION('center_axis',(1.,0.,0.));
#5436=DIRECTION('ref_axis',(0.,0.,-1.));
#5437=DIRECTION('center_axis',(1.,0.,0.));
#5438=DIRECTION('ref_axis',(0.,1.,0.));
#5439=DIRECTION('center_axis',(1.,0.,0.));
#5440=DIRECTION('ref_axis',(0.,0.,-1.));
#5441=DIRECTION('',(1.,0.,0.));
#5442=DIRECTION('center_axis',(-1.,0.,0.));
#5443=DIRECTION('ref_axis',(0.,0.,1.));
#5444=DIRECTION('center_axis',(-1.,0.,0.));
#5445=DIRECTION('ref_axis',(0.,1.,0.));
#5446=DIRECTION('center_axis',(1.,0.,0.));
#5447=DIRECTION('ref_axis',(0.,1.,0.));
#5448=DIRECTION('',(-1.,0.,0.));
#5449=DIRECTION('center_axis',(1.,0.,0.));
#5450=DIRECTION('ref_axis',(0.,1.,0.));
#5451=DIRECTION('center_axis',(1.,0.,0.));
#5452=DIRECTION('ref_axis',(0.,0.,-1.));
#5453=DIRECTION('center_axis',(1.,0.,0.));
#5454=DIRECTION('ref_axis',(0.,0.,-1.));
#5455=DIRECTION('center_axis',(1.,0.,0.));
#5456=DIRECTION('ref_axis',(0.,1.,0.));
#5457=DIRECTION('center_axis',(1.,0.,0.));
#5458=DIRECTION('ref_axis',(0.,0.,-1.));
#5459=DIRECTION('',(1.,0.,0.));
#5460=DIRECTION('center_axis',(-1.,0.,0.));
#5461=DIRECTION('ref_axis',(0.,0.,1.));
#5462=DIRECTION('center_axis',(-1.,0.,0.));
#5463=DIRECTION('ref_axis',(0.,1.,0.));
#5464=DIRECTION('center_axis',(1.,0.,0.));
#5465=DIRECTION('ref_axis',(0.,1.,0.));
#5466=DIRECTION('',(-1.,0.,0.));
#5467=DIRECTION('center_axis',(1.,0.,0.));
#5468=DIRECTION('ref_axis',(0.,0.,-1.));
#5469=DIRECTION('center_axis',(-1.,0.,0.));
#5470=DIRECTION('ref_axis',(0.,0.,1.));
#5471=DIRECTION('center_axis',(1.,0.,0.));
#5472=DIRECTION('ref_axis',(0.,0.,-1.));
#5473=DIRECTION('center_axis',(1.,0.,0.));
#5474=DIRECTION('ref_axis',(0.,1.,0.));
#5475=DIRECTION('',(-0.707106781186547,0.707106781186548,8.65956056235494E-17));
#5476=DIRECTION('center_axis',(1.,0.,0.));
#5477=DIRECTION('ref_axis',(0.,1.,0.));
#5478=DIRECTION('center_axis',(1.,0.,0.));
#5479=DIRECTION('ref_axis',(0.,0.,-1.));
#5480=DIRECTION('',(-1.,0.,0.));
#5481=DIRECTION('center_axis',(-1.,0.,0.));
#5482=DIRECTION('ref_axis',(0.,1.,0.));
#5483=DIRECTION('center_axis',(1.,0.,0.));
#5484=DIRECTION('ref_axis',(0.,0.,-1.));
#5485=DIRECTION('',(-0.707106781186556,-0.707106781186539,-8.65956056235483E-17));
#5486=DIRECTION('center_axis',(1.,0.,0.));
#5487=DIRECTION('ref_axis',(0.,0.,-1.));
#7731=CARTESIAN_POINT('',(0.,0.,0.));
#7732=CARTESIAN_POINT('Origin',(84.65,0.,0.));
#7733=CARTESIAN_POINT('',(92.9209088298366,-3.45967356244292,-0.00100989411776997));
#7734=CARTESIAN_POINT('',(93.2183732864721,-3.44877006476889,0.000221723780192462));
#7735=CARTESIAN_POINT('',(84.65,-3.4544,-4.23041990297462E-16));
#7736=CARTESIAN_POINT('',(93.8044,3.25944077490411,1.14408268708712));
#7737=CARTESIAN_POINT('Ctrl Pts',(93.2183732864721,-3.44877006476889,0.000221723780192462));
#7738=CARTESIAN_POINT('Ctrl Pts',(93.2462262172957,-3.448754724225,-0.573040469566619));
#7739=CARTESIAN_POINT('Ctrl Pts',(93.2740791481193,-3.31345071435984,-1.14634497961049));
#7740=CARTESIAN_POINT('Ctrl Pts',(93.3019320789429,-3.04283652130647,-1.64659870953629));
#7741=CARTESIAN_POINT('Ctrl Pts',(93.3577618479492,-2.50040427301956,-2.64933161269944));
#7742=CARTESIAN_POINT('Ctrl Pts',(93.4135916169555,-1.41432083486459,-3.35856004638195));
#7743=CARTESIAN_POINT('Ctrl Pts',(93.4694213859618,-0.277922290246916,-3.44943135077171));
#7744=CARTESIAN_POINT('Ctrl Pts',(93.5252511549682,0.858476254370759,-3.54030265516147));
#7745=CARTESIAN_POINT('Ctrl Pts',(93.5810809239746,2.04518990545115,-3.01281683025845));
#7746=CARTESIAN_POINT('Ctrl Pts',(93.636910692981,2.74023372258513,-2.11180914044543));
#7747=CARTESIAN_POINT('Ctrl Pts',(93.6927404619873,3.43527753971911,-1.21080145063241));
#7748=CARTESIAN_POINT('Ctrl Pts',(93.7485702309937,3.6386515229067,0.063728104090605));
#7749=CARTESIAN_POINT('Ctrl Pts',(93.8044,3.25944077490411,1.14408268708712));
#7750=CARTESIAN_POINT('',(93.8044,-1.75208009336914,2.97731016051328));
#7751=CARTESIAN_POINT('Origin',(93.8044,0.,0.));
#7752=CARTESIAN_POINT('Ctrl Pts',(93.8044,-1.75208009336914,2.97731016051328));
#7753=CARTESIAN_POINT('Ctrl Pts',(93.7917271656399,-1.52951455720307,3.11157965083414));
#7754=CARTESIAN_POINT('Ctrl Pts',(93.7790543312797,-1.2925249415104,3.22041651535433));
#7755=CARTESIAN_POINT('Ctrl Pts',(93.7663814969195,-1.04589844408296,3.2987746062456));
#7756=CARTESIAN_POINT('Ctrl Pts',(93.7105517279132,0.0406067520640256,3.64397868529463));
#7757=CARTESIAN_POINT('Ctrl Pts',(93.6547219589068,1.31414599657454,3.39764614722317));
#7758=CARTESIAN_POINT('Ctrl Pts',(93.5988921899005,2.19521568785426,2.67416693511821));
#7759=CARTESIAN_POINT('Ctrl Pts',(93.5430624208941,3.07628537913397,1.95068772301326));
#7760=CARTESIAN_POINT('Ctrl Pts',(93.4872326518878,3.56488551718289,0.750061836874816));
#7761=CARTESIAN_POINT('Ctrl Pts',(93.4314028828814,3.43877773600297,-0.382618805547265));
#7762=CARTESIAN_POINT('Ctrl Pts',(93.3755731138751,3.31266995482305,-1.51529944796938));
#7763=CARTESIAN_POINT('Ctrl Pts',(93.3197433448686,2.57185425441423,-2.58003484667512));
#7764=CARTESIAN_POINT('Ctrl Pts',(93.2639135758623,1.55334430498576,-3.09183132689595));
#7765=CARTESIAN_POINT('Ctrl Pts',(93.2080838068559,0.534834355557293,-3.60362780711678));
#7766=CARTESIAN_POINT('Ctrl Pts',(93.1522540378496,-0.761369842890835,-3.5624853688527));
#7767=CARTESIAN_POINT('Ctrl Pts',(93.0964242688433,-1.74552965897778,-2.98741603452504));
#7768=CARTESIAN_POINT('Ctrl Pts',(93.0405944998369,-2.72968947506471,-2.41234670019739));
#7769=CARTESIAN_POINT('Ctrl Pts',(92.9847647308305,-3.40180490879047,-1.30335046980618));
#7770=CARTESIAN_POINT('Ctrl Pts',(92.9289349618241,-3.45609656090976,-0.164829487232134));
#7771=CARTESIAN_POINT('Ctrl Pts',(92.9262595844949,-3.45869823127002,-0.110271259967334));
#7772=CARTESIAN_POINT('Ctrl Pts',(92.9235842071657,-3.45988116087502,-0.0556452334846064));
#7773=CARTESIAN_POINT('Ctrl Pts',(92.9209088298366,-3.45967356244292,-0.00100989411776997));
#7774=CARTESIAN_POINT('Origin',(84.65,0.,0.));
#7775=CARTESIAN_POINT('',(91.8625754965033,-3.45043530540852,-0.00223112594461949));
#7776=CARTESIAN_POINT('',(92.1600399531387,-3.45616980202756,0.00289452556765842));
#7777=CARTESIAN_POINT('',(84.65,-3.4544,-4.23041990297462E-16));
#7778=CARTESIAN_POINT('Ctrl Pts',(92.1600399531387,-3.45616980202756,0.00289452556765842));
#7779=CARTESIAN_POINT('Ctrl Pts',(92.2056920477019,-3.44779680921498,-0.931879971447121));
#7780=CARTESIAN_POINT('Ctrl Pts',(92.2513441422651,-3.05497186656688,-1.87285172139297));
#7781=CARTESIAN_POINT('Ctrl Pts',(92.2969962368283,-2.37792145309273,-2.51340958946608));
#7782=CARTESIAN_POINT('Ctrl Pts',(92.3528260058347,-1.54992947262409,-3.29677337927473));
#7783=CARTESIAN_POINT('Ctrl Pts',(92.408655774841,-0.296854978392081,-3.63084355825839));
#7784=CARTESIAN_POINT('Ctrl Pts',(92.4644855438474,0.811213403585058,-3.36359464588894));
#7785=CARTESIAN_POINT('Ctrl Pts',(92.5203153128537,1.91928178556216,-3.0963457335195));
#7786=CARTESIAN_POINT('Ctrl Pts',(92.5761450818601,2.88234405528443,-2.22777772979697));
#7787=CARTESIAN_POINT('Ctrl Pts',(92.6319748508664,3.26221848023226,-1.15312751939853));
#7788=CARTESIAN_POINT('Ctrl Pts',(92.6878046198728,3.6420929051801,-0.0784773090000682));
#7789=CARTESIAN_POINT('Ctrl Pts',(92.7436343888792,3.43877948535351,1.20225510807429));
#7790=CARTESIAN_POINT('Ctrl Pts',(92.7994641578856,2.74482734879403,2.10652594559603));
#7791=CARTESIAN_POINT('Ctrl Pts',(92.855293926892,2.05087521223453,3.0107967831178));
#7792=CARTESIAN_POINT('Ctrl Pts',(92.9111236958982,0.86628435894208,3.53860604108688));
#7793=CARTESIAN_POINT('Ctrl Pts',(92.9669534649046,-0.270098466384267,3.44954294338115));
#7794=CARTESIAN_POINT('Ctrl Pts',(93.0227832339109,-1.40648129171058,3.36047984567542));
#7795=CARTESIAN_POINT('Ctrl Pts',(93.0786130029174,-2.49465608907082,2.65454439229492));
#7796=CARTESIAN_POINT('Ctrl Pts',(93.1344427719237,-3.03935295854151,1.65345797928278));
#7797=CARTESIAN_POINT('Ctrl Pts',(93.1624196101066,-3.31230583739212,1.15180387821292));
#7798=CARTESIAN_POINT('Ctrl Pts',(93.1903964482893,-3.44878547355717,0.576034148015107));
#7799=CARTESIAN_POINT('Ctrl Pts',(93.2183732864721,-3.44877006476889,0.000221723780192462));
#7800=CARTESIAN_POINT('Ctrl Pts',(92.9209088298366,-3.45967356244292,-0.00100989411776997));
#7801=CARTESIAN_POINT('Ctrl Pts',(92.8677544381594,-3.45554899718949,1.08448492428777));
#7802=CARTESIAN_POINT('Ctrl Pts',(92.8146000464823,-2.902531081883,2.17365588587066));
#7803=CARTESIAN_POINT('Ctrl Pts',(92.7614456548051,-2.02188203340776,2.80781567790935));
#7804=CARTESIAN_POINT('Ctrl Pts',(92.7056158857987,-1.09690798327364,3.47389412571991));
#7805=CARTESIAN_POINT('Ctrl Pts',(92.6497861167924,0.189507987507439,3.63800528658412));
#7806=CARTESIAN_POINT('Ctrl Pts',(92.593956347786,1.25209352043107,3.22552316675482));
#7807=CARTESIAN_POINT('Ctrl Pts',(92.5381265787796,2.31467905335469,2.81304104692552));
#7808=CARTESIAN_POINT('Ctrl Pts',(92.4822968097733,3.15343414842088,1.82396564640271));
#7809=CARTESIAN_POINT('Ctrl Pts',(92.4264670407669,3.38675808805357,0.708269247798187));
#7810=CARTESIAN_POINT('Ctrl Pts',(92.3706372717606,3.62008202768626,-0.407427150806336));
#7811=CARTESIAN_POINT('Ctrl Pts',(92.3148075027542,3.24797481188544,-1.64974454749257));
#7812=CARTESIAN_POINT('Ctrl Pts',(92.2589777337479,2.43973058675324,-2.45346584442737));
#7813=CARTESIAN_POINT('Ctrl Pts',(92.2031479647415,1.63148636162103,-3.25718714136217));
#7814=CARTESIAN_POINT('Ctrl Pts',(92.1473181957351,0.387105127157411,-3.62231233854551));
#7815=CARTESIAN_POINT('Ctrl Pts',(92.0914884267288,-0.727266665982812,-3.38272834733937));
#7816=CARTESIAN_POINT('Ctrl Pts',(92.0356586577225,-1.84163845912302,-3.14314435613323));
#7817=CARTESIAN_POINT('Ctrl Pts',(91.9798288887161,-2.82600081093984,-2.29885117653763));
#7818=CARTESIAN_POINT('Ctrl Pts',(91.9239991197097,-3.23250637058094,-1.23396759562083));
#7819=CARTESIAN_POINT('Ctrl Pts',(91.9035245786409,-3.38158480890701,-0.843441125620498));
#7820=CARTESIAN_POINT('Ctrl Pts',(91.8830500375721,-3.45294608894601,-0.423246995105974));
#7821=CARTESIAN_POINT('Ctrl Pts',(91.8625754965033,-3.45043530540852,-0.00223112594461949));
#7822=CARTESIAN_POINT('Origin',(84.65,0.,0.));
#7823=CARTESIAN_POINT('',(90.80424216317,-3.45180239605614,0.00279451803522027));
#7824=CARTESIAN_POINT('',(91.1017066198054,-3.45763635249975,-0.00244580608254598));
#7825=CARTESIAN_POINT('',(84.65,-3.4544,-4.23041990297462E-16));
#7826=CARTESIAN_POINT('Ctrl Pts',(91.1017066198054,-3.45763635249975,-0.00244580608254598));
#7827=CARTESIAN_POINT('Ctrl Pts',(91.1093281091019,-3.45888988877411,-0.158332497209808));
#7828=CARTESIAN_POINT('Ctrl Pts',(91.1169495983983,-3.44925346319397,-0.314063335739518));
#7829=CARTESIAN_POINT('Ctrl Pts',(91.1245710876948,-3.428196288038,-0.468234288642407));
#7830=CARTESIAN_POINT('Ctrl Pts',(91.1804008567011,-3.27394595989943,-1.59758425598427));
#7831=CARTESIAN_POINT('Ctrl Pts',(91.2362306257075,-2.50685636728464,-2.64323050897187));
#7832=CARTESIAN_POINT('Ctrl Pts',(91.2920603947139,-1.47592424748071,-3.12944403336781));
#7833=CARTESIAN_POINT('Ctrl Pts',(91.3478901637202,-0.444992127676794,-3.61565755776375));
#7834=CARTESIAN_POINT('Ctrl Pts',(91.4037199327265,0.849782519316258,-3.54243835356805));
#7835=CARTESIAN_POINT('Ctrl Pts',(91.4595497017329,1.81932662547287,-2.94309775990678));
#7836=CARTESIAN_POINT('Ctrl Pts',(91.5153794707393,2.78887073162951,-2.3437571662455));
#7837=CARTESIAN_POINT('Ctrl Pts',(91.5712092397457,3.43318429694969,-1.21829518311862));
#7838=CARTESIAN_POINT('Ctrl Pts',(91.6270390087521,3.45912869688117,-0.0787554811289303));
#7839=CARTESIAN_POINT('Ctrl Pts',(91.6828687777584,3.48507309681266,1.06078422086078));
#7840=CARTESIAN_POINT('Ctrl Pts',(91.7386985467648,2.89264833135546,2.21440164171326));
#7841=CARTESIAN_POINT('Ctrl Pts',(91.7945283157711,1.9513860055696,2.85724707365223));
#7842=CARTESIAN_POINT('Ctrl Pts',(91.8503580847774,1.01012367978377,3.50009250559118));
#7843=CARTESIAN_POINT('Ctrl Pts',(91.9061878537838,-0.279976206330739,3.6321659486166));
#7844=CARTESIAN_POINT('Ctrl Pts',(91.9620176227901,-1.33196886180909,3.19337427179059));
#7845=CARTESIAN_POINT('Ctrl Pts',(92.0178473917965,-2.38396151728742,2.75458259496459));
#7846=CARTESIAN_POINT('Ctrl Pts',(92.0736771608029,-3.19784694212965,1.7449257982872));
#7847=CARTESIAN_POINT('Ctrl Pts',(92.1295069298093,-3.40333492119814,0.623768699631705));
#7848=CARTESIAN_POINT('Ctrl Pts',(92.1396846042524,-3.44079503952147,0.419383617034329));
#7849=CARTESIAN_POINT('Ctrl Pts',(92.1498622786956,-3.45803647639982,0.211293079881917));
#7850=CARTESIAN_POINT('Ctrl Pts',(92.1600399531387,-3.45616980202756,0.00289452556765842));
#7851=CARTESIAN_POINT('Ctrl Pts',(91.8625754965033,-3.45043530540852,-0.00223112594461949));
#7852=CARTESIAN_POINT('Ctrl Pts',(91.8272202685657,-3.44609971009669,0.724774767349627));
#7853=CARTESIAN_POINT('Ctrl Pts',(91.7918650406282,-3.22149218222548,1.45423092331462));
#7854=CARTESIAN_POINT('Ctrl Pts',(91.7565098126906,-2.7964109095389,2.03761122757244));
#7855=CARTESIAN_POINT('Ctrl Pts',(91.7006800436842,-2.12516112139035,2.95883248761094));
#7856=CARTESIAN_POINT('Ctrl Pts',(91.6448502746779,-0.954012777627767,3.51580102544994));
#7857=CARTESIAN_POINT('Ctrl Pts',(91.5890205056715,0.184206076595443,3.45511796588552));
#7858=CARTESIAN_POINT('Ctrl Pts',(91.5331907366652,1.32242493081865,3.3944349063211));
#7859=CARTESIAN_POINT('Ctrl Pts',(91.4773609676588,2.42771429550253,2.71610024935329));
#7860=CARTESIAN_POINT('Ctrl Pts',(91.4215311986524,2.99720950963122,1.72873016655719));
#7861=CARTESIAN_POINT('Ctrl Pts',(91.3657014296461,3.56670472375992,0.741360083761087));
#7862=CARTESIAN_POINT('Ctrl Pts',(91.3098716606398,3.60040578733339,-0.555045424863321));
#7863=CARTESIAN_POINT('Ctrl Pts',(91.2540418916334,3.08297998794191,-1.57067092694823));
#7864=CARTESIAN_POINT('Ctrl Pts',(91.198212122627,2.56555418855044,-2.58629642903311));
#7865=CARTESIAN_POINT('Ctrl Pts',(91.1423823536206,1.49700152619402,-3.32114192457851));
#7866=CARTESIAN_POINT('Ctrl Pts',(91.0865525846143,0.363472878981578,-3.44088071064219));
#7867=CARTESIAN_POINT('Ctrl Pts',(91.0307228156079,-0.770055768230898,-3.56061949670588));
#7868=CARTESIAN_POINT('Ctrl Pts',(90.9748930466016,-1.9685604002994,-3.06525157328782));
#7869=CARTESIAN_POINT('Ctrl Pts',(90.9190632775953,-2.68676693551405,-2.18015048631885));
#7870=CARTESIAN_POINT('Ctrl Pts',(90.8807895727868,-3.1791283657962,-1.57337567189296));
#7871=CARTESIAN_POINT('Ctrl Pts',(90.8425158679784,-3.44576451119845,-0.783438296661764));
#7872=CARTESIAN_POINT('Ctrl Pts',(90.80424216317,-3.45180239605614,0.00279451803522027));
#7873=CARTESIAN_POINT('Origin',(84.65,0.,0.));
#7874=CARTESIAN_POINT('',(89.7459088298366,-3.46002183154878,-9.14716326361198E-5));
#7875=CARTESIAN_POINT('',(90.043373286472,-3.44903894306056,-0.000821802180914491));
#7876=CARTESIAN_POINT('',(84.65,-3.4544,-4.23041990297462E-16));
#7877=CARTESIAN_POINT('Ctrl Pts',(90.043373286472,-3.44903894306056,-0.000821802180914491));
#7878=CARTESIAN_POINT('Ctrl Pts',(90.0687939395081,-3.45015973575754,-0.524074439861875));
#7879=CARTESIAN_POINT('Ctrl Pts',(90.0942145925442,-3.33844059682494,-1.04687294234206));
#7880=CARTESIAN_POINT('Ctrl Pts',(90.1196352455803,-3.11140810631006,-1.51357609271899));
#7881=CARTESIAN_POINT('Ctrl Pts',(90.1754650145866,-2.61279103756708,-2.5385666404873));
#7882=CARTESIAN_POINT('Ctrl Pts',(90.2312947835931,-1.55796517491713,-3.29298376627957));
#7883=CARTESIAN_POINT('Ctrl Pts',(90.2871245525994,-0.426836221514585,-3.43359633877573));
#7884=CARTESIAN_POINT('Ctrl Pts',(90.3429543216058,0.704292731887955,-3.57420891127189));
#7885=CARTESIAN_POINT('Ctrl Pts',(90.3987840906121,1.91172477604308,-3.10101693047194));
#7886=CARTESIAN_POINT('Ctrl Pts',(90.4546138596185,2.64612419731206,-2.22930476351716));
#7887=CARTESIAN_POINT('Ctrl Pts',(90.5104436286248,3.38052361858102,-1.35759259656241));
#7888=CARTESIAN_POINT('Ctrl Pts',(90.5662733976312,3.64189041696387,-0.0873602434528473));
#7889=CARTESIAN_POINT('Ctrl Pts',(90.6221031666375,3.31131261962515,1.0034848025557));
#7890=CARTESIAN_POINT('Ctrl Pts',(90.6779329356439,2.98073482228642,2.09432984856429));
#7891=CARTESIAN_POINT('Ctrl Pts',(90.7337627046502,2.05821242922608,3.00578758747185));
#7892=CARTESIAN_POINT('Ctrl Pts',(90.7895924736566,0.963458102751407,3.32317940954435));
#7893=CARTESIAN_POINT('Ctrl Pts',(90.845422242663,-0.131296223723232,3.64057123161685));
#7894=CARTESIAN_POINT('Ctrl Pts',(90.9012520116694,-1.39828248361219,3.36389713685432));
#7895=CARTESIAN_POINT('Ctrl Pts',(90.9570817806757,-2.26107008172552,2.61903324862501));
#7896=CARTESIAN_POINT('Ctrl Pts',(91.0052900603856,-3.00607595583795,1.97585296490451));
#7897=CARTESIAN_POINT('Ctrl Pts',(91.0534983400955,-3.44970734742079,0.983585783884964));
#7898=CARTESIAN_POINT('Ctrl Pts',(91.1017066198054,-3.45763635249975,-0.00244580608254598));
#7899=CARTESIAN_POINT('Ctrl Pts',(90.80424216317,-3.45180239605614,0.00279451803522027));
#7900=CARTESIAN_POINT('Ctrl Pts',(90.786686098972,-3.45457196055772,0.363437780515883));
#7901=CARTESIAN_POINT('Ctrl Pts',(90.7691300347741,-3.40251069416784,0.723301589857626));
#7902=CARTESIAN_POINT('Ctrl Pts',(90.7515739705762,-3.29225294667203,1.06435108224323));
#7903=CARTESIAN_POINT('Ctrl Pts',(90.6957442015698,-2.9416239842546,2.14891731331652));
#7904=CARTESIAN_POINT('Ctrl Pts',(90.6399144325634,-2.00245762105894,3.04321552494328));
#7905=CARTESIAN_POINT('Ctrl Pts',(90.584084663557,-0.902038879867245,3.34037401075845));
#7906=CARTESIAN_POINT('Ctrl Pts',(90.5282548945507,0.198379861324493,3.63753249657364));
#7907=CARTESIAN_POINT('Ctrl Pts',(90.4724251255444,1.46005098051228,3.33755125657718));
#7908=CARTESIAN_POINT('Ctrl Pts',(90.416595356538,2.30896204172667,2.57691035490764));
#7909=CARTESIAN_POINT('Ctrl Pts',(90.3607655875317,3.15787310294103,1.81626945323814));
#7910=CARTESIAN_POINT('Ctrl Pts',(90.3049358185253,3.59402410618203,0.594968889895604));
#7911=CARTESIAN_POINT('Ctrl Pts',(90.2491060495189,3.41898291147,-0.53134596547945));
#7912=CARTESIAN_POINT('Ctrl Pts',(90.1932762805125,3.24394171675795,-1.65766082085454));
#7913=CARTESIAN_POINT('Ctrl Pts',(90.1374465115062,2.45770832409283,-2.68898996826213));
#7914=CARTESIAN_POINT('Ctrl Pts',(90.0816167424998,1.41798906313595,-3.15611782081291));
#7915=CARTESIAN_POINT('Ctrl Pts',(90.0257869734935,0.378269802179101,-3.62324567336368));
#7916=CARTESIAN_POINT('Ctrl Pts',(89.9699572044871,-0.914935327069492,-3.52617223105767));
#7917=CARTESIAN_POINT('Ctrl Pts',(89.9141274354808,-1.87326711159148,-2.90906222219465));
#7918=CARTESIAN_POINT('Ctrl Pts',(89.8582976664744,-2.83159889611351,-2.29195221333161));
#7919=CARTESIAN_POINT('Ctrl Pts',(89.802467897468,-3.4550573359089,-1.15480563791153));
#7920=CARTESIAN_POINT('Ctrl Pts',(89.7466381284617,-3.45999252212756,-0.0149809950586317));
#7921=CARTESIAN_POINT('Ctrl Pts',(89.74639502892,-3.46001401140702,-0.0100178570549767));
#7922=CARTESIAN_POINT('Ctrl Pts',(89.7461519293783,-3.46002377353189,-0.00505466827536287));
#7923=CARTESIAN_POINT('Ctrl Pts',(89.7459088298366,-3.46002183154878,-9.14716326361198E-5));
#7924=CARTESIAN_POINT('Origin',(84.65,0.,0.));
#7925=CARTESIAN_POINT('',(88.6875754965033,-3.45155207576766,-0.00271849840084493));
#7926=CARTESIAN_POINT('',(88.9850399531387,-3.454679949607,0.00309179818855912));
#7927=CARTESIAN_POINT('',(84.65,-3.4544,-4.23041990297462E-16));
#7928=CARTESIAN_POINT('Ctrl Pts',(88.9850399531387,-3.454679949607,0.00309179818855912));
#7929=CARTESIAN_POINT('Ctrl Pts',(89.0282597699144,-3.44660062115878,-0.88286530776684));
#7930=CARTESIAN_POINT('Ctrl Pts',(89.0714795866901,-3.09865605805359,-1.77446071433409));
#7931=CARTESIAN_POINT('Ctrl Pts',(89.1146994034658,-2.48454027584772,-2.40807653662655));
#7932=CARTESIAN_POINT('Ctrl Pts',(89.1705291724722,-1.6912481052297,-3.2265581415103));
#7933=CARTESIAN_POINT('Ctrl Pts',(89.2263589414785,-0.453808750692432,-3.61456155175139));
#7934=CARTESIAN_POINT('Ctrl Pts',(89.2821887104849,0.664789883977839,-3.3955599535972));
#7935=CARTESIAN_POINT('Ctrl Pts',(89.3380184794913,1.78338851864816,-3.176558355443));
#7936=CARTESIAN_POINT('Ctrl Pts',(89.3938482484977,2.78314643345148,-2.35055174889353));
#7937=CARTESIAN_POINT('Ctrl Pts',(89.449678017504,3.20921175174797,-1.2933417649389));
#7938=CARTESIAN_POINT('Ctrl Pts',(89.5055077865104,3.63527707004444,-0.236131780984317));
#7939=CARTESIAN_POINT('Ctrl Pts',(89.5613375555167,3.48764979183407,1.05228158037541));
#7940=CARTESIAN_POINT('Ctrl Pts',(89.617167324523,2.8334947211445,1.98571917811078));
#7941=CARTESIAN_POINT('Ctrl Pts',(89.6729970935294,2.17933965045492,2.91915677584617));
#7942=CARTESIAN_POINT('Ctrl Pts',(89.7288268625358,1.01865678728613,3.49761860995722));
#7943=CARTESIAN_POINT('Ctrl Pts',(89.7846566315421,-0.120487252438666,3.45792651875769));
#7944=CARTESIAN_POINT('Ctrl Pts',(89.8404864005485,-1.25963129216346,3.41823442755817));
#7945=CARTESIAN_POINT('Ctrl Pts',(89.8963161695549,-2.37723650844425,2.76038841104806));
#7946=CARTESIAN_POINT('Ctrl Pts',(89.9521459385612,-2.96483497916664,1.78368341792084));
#7947=CARTESIAN_POINT('Ctrl Pts',(89.9825550545315,-3.28488556075007,1.25169598660317));
#7948=CARTESIAN_POINT('Ctrl Pts',(90.0129641705018,-3.44769820979724,0.625112162552654));
#7949=CARTESIAN_POINT('Ctrl Pts',(90.043373286472,-3.44903894306056,-0.000821802180914491));
#7950=CARTESIAN_POINT('Ctrl Pts',(89.7459088298366,-3.46002183154878,-9.14716326361198E-5));
#7951=CARTESIAN_POINT('Ctrl Pts',(89.6903221603719,-3.45957778145935,1.13478344151281));
#7952=CARTESIAN_POINT('Ctrl Pts',(89.6347354909072,-2.8471902022148,2.27006947366597));
#7953=CARTESIAN_POINT('Ctrl Pts',(89.5791488214426,-1.89838758434876,2.8927317993208));
#7954=CARTESIAN_POINT('Ctrl Pts',(89.5233190524362,-0.945435527709273,3.51811724056172));
#7955=CARTESIAN_POINT('Ctrl Pts',(89.4674892834298,0.346880518211697,3.62638541275787));
#7956=CARTESIAN_POINT('Ctrl Pts',(89.4116595144235,1.39060583950645,3.16827840989243));
#7957=CARTESIAN_POINT('Ctrl Pts',(89.3558297454172,2.43433116080121,2.710171407027));
#7958=CARTESIAN_POINT('Ctrl Pts',(89.2999999764108,3.22946575746975,1.68568922909996));
#7959=CARTESIAN_POINT('Ctrl Pts',(89.2441702074045,3.41425359020177,0.560932353464458));
#7960=CARTESIAN_POINT('Ctrl Pts',(89.1883404383981,3.59904142293379,-0.563824522171029));
#7961=CARTESIAN_POINT('Ctrl Pts',(89.1325106693917,3.1734824917293,-1.78885609551498));
#7962=CARTESIAN_POINT('Ctrl Pts',(89.0766809003854,2.33118994597285,-2.55681953198702));
#7963=CARTESIAN_POINT('Ctrl Pts',(89.020851131379,1.4888974002164,-3.32478296845905));
#7964=CARTESIAN_POINT('Ctrl Pts',(88.9650213623726,0.229871239907982,-3.63567826805917));
#7965=CARTESIAN_POINT('Ctrl Pts',(88.9091915933663,-0.873079454520174,-3.34805987841929));
#7966=CARTESIAN_POINT('Ctrl Pts',(88.8533618243599,-1.97603014894834,-3.0604414887794));
#7967=CARTESIAN_POINT('Ctrl Pts',(88.7975320553536,-2.92290537749625,-2.17430940989949));
#7968=CARTESIAN_POINT('Ctrl Pts',(88.7417022863472,-3.28291287702557,-1.09282007907629));
#7969=CARTESIAN_POINT('Ctrl Pts',(88.7236600230659,-3.39925493262351,-0.743319882497822));
#7970=CARTESIAN_POINT('Ctrl Pts',(88.7056177597846,-3.45430685025923,-0.373417349359545));
#7971=CARTESIAN_POINT('Ctrl Pts',(88.6875754965033,-3.45155207576766,-0.00271849840084493));
#7972=CARTESIAN_POINT('Origin',(84.65,0.,0.));
#7973=CARTESIAN_POINT('',(87.6292421631699,-3.45063882513586,0.00234158759808215));
#7974=CARTESIAN_POINT('',(87.9267066198054,-3.45881529047273,-0.00181033228093454));
#7975=CARTESIAN_POINT('',(84.65,-3.4544,-4.23041990297462E-16));
#7976=CARTESIAN_POINT('Ctrl Pts',(87.9267066198054,-3.45881529047273,-0.00181033228093454));
#7977=CARTESIAN_POINT('Ctrl Pts',(87.9318958313143,-3.45949248446936,-0.107853322368814));
#7978=CARTESIAN_POINT('Ctrl Pts',(87.9370850428233,-3.45503548807332,-0.213838636952292));
#7979=CARTESIAN_POINT('Ctrl Pts',(87.9422742543323,-3.44525773166627,-0.319330785970636));
#7980=CARTESIAN_POINT('Ctrl Pts',(87.9981040233386,-3.34006065487291,-1.45430134970563));
#7981=CARTESIAN_POINT('Ctrl Pts',(88.053933792345,-2.61897437949145,-2.53218695864979));
#7982=CARTESIAN_POINT('Ctrl Pts',(88.1097635613514,-1.61006577127509,-3.06259060284673));
#7983=CARTESIAN_POINT('Ctrl Pts',(88.1655933303578,-0.601157163058717,-3.59299424704368));
#7984=CARTESIAN_POINT('Ctrl Pts',(88.2214230993641,0.695573777992526,-3.57591592649341));
#7985=CARTESIAN_POINT('Ctrl Pts',(88.2772528683704,1.69016372837544,-3.01912562834955));
#7986=CARTESIAN_POINT('Ctrl Pts',(88.3330826373768,2.68475367875835,-2.46233533020569));
#7987=CARTESIAN_POINT('Ctrl Pts',(88.3889124063832,3.37720263847291,-1.36583305446821));
#7988=CARTESIAN_POINT('Ctrl Pts',(88.4447421753896,3.45247263264309,-0.228485687350275));
#7989=CARTESIAN_POINT('Ctrl Pts',(88.5005719443959,3.52774262681328,0.908861679767659));
#7990=CARTESIAN_POINT('Ctrl Pts',(88.5564017134023,2.98583365543915,2.08705413826606));
#7991=CARTESIAN_POINT('Ctrl Pts',(88.6122314824086,2.07329371677074,2.77005887166429));
#7992=CARTESIAN_POINT('Ctrl Pts',(88.668061251415,1.16075377810231,3.45306360506253));
#7993=CARTESIAN_POINT('Ctrl Pts',(88.7238910204213,-0.122417127860435,3.64088061336055));
#7994=CARTESIAN_POINT('Ctrl Pts',(88.7797207894276,-1.19242497851517,3.24806029178481));
#7995=CARTESIAN_POINT('Ctrl Pts',(88.835550558434,-2.26243282916989,2.85523997020907));
#7996=CARTESIAN_POINT('Ctrl Pts',(88.8913803274404,-3.11927762451663,1.88178231875958));
#7997=CARTESIAN_POINT('Ctrl Pts',(88.9472100964468,-3.37312752884059,0.770573593271612));
#7998=CARTESIAN_POINT('Ctrl Pts',(88.9598200486774,-3.43046316221776,0.519591201689593));
#7999=CARTESIAN_POINT('Ctrl Pts',(88.9724300009081,-3.45703720036345,0.261581482272195));
#8000=CARTESIAN_POINT('Ctrl Pts',(88.9850399531387,-3.454679949607,0.00309179818855912));
#8001=CARTESIAN_POINT('Ctrl Pts',(88.6875754965033,-3.45155207576766,-0.00271849840084493));
#8002=CARTESIAN_POINT('Ctrl Pts',(88.6497879907782,-3.44578250821131,0.773668850262181));
#8003=CARTESIAN_POINT('Ctrl Pts',(88.6120004850532,-3.18644605389839,1.55354921717556));
#8004=CARTESIAN_POINT('Ctrl Pts',(88.5742129793281,-2.7055449759783,2.15680297346112));
#8005=CARTESIAN_POINT('Ctrl Pts',(88.5183832103217,-1.99502980489096,3.04809011240894));
#8006=CARTESIAN_POINT('Ctrl Pts',(88.4625534413154,-0.800859692205512,3.55381780753807));
#8007=CARTESIAN_POINT('Ctrl Pts',(88.4067236723091,0.333663319839212,3.44389916698642));
#8008=CARTESIAN_POINT('Ctrl Pts',(88.3508939033027,1.46818633188394,3.33398052643478));
#8009=CARTESIAN_POINT('Ctrl Pts',(88.2950641342964,2.54306224328792,2.60841555020236));
#8010=CARTESIAN_POINT('Ctrl Pts',(88.23923436529,3.06926334215677,1.59730874281291));
#8011=CARTESIAN_POINT('Ctrl Pts',(88.1834045962837,3.59546444102562,0.586201935423477));
#8012=CARTESIAN_POINT('Ctrl Pts',(88.1275748272773,3.57299072735933,-0.710446703122968));
#8013=CARTESIAN_POINT('Ctrl Pts',(88.0717450582709,3.01206688724067,-1.70271129383767));
#8014=CARTESIAN_POINT('Ctrl Pts',(88.0159152892645,2.45114304712202,-2.69497588455235));
#8015=CARTESIAN_POINT('Ctrl Pts',(87.9600855202581,1.35176908055096,-3.38285642743532));
#8016=CARTESIAN_POINT('Ctrl Pts',(87.9042557512518,0.214118383995447,-3.45339340374213));
#8017=CARTESIAN_POINT('Ctrl Pts',(87.8484259822454,-0.923532312560085,-3.52393038004894));
#8018=CARTESIAN_POINT('Ctrl Pts',(87.7925962132391,-2.0994597391001,-2.97712378977962));
#8019=CARTESIAN_POINT('Ctrl Pts',(87.7367664442328,-2.77866158265664,-2.06174986175392));
#8020=CARTESIAN_POINT('Ctrl Pts',(87.7009250172118,-3.21469353732137,-1.47410086334105));
#8021=CARTESIAN_POINT('Ctrl Pts',(87.6650835901909,-3.446007764652,-0.734552566120437));
#8022=CARTESIAN_POINT('Ctrl Pts',(87.6292421631699,-3.45063882513586,0.00234158759808215));
#8023=CARTESIAN_POINT('Origin',(84.65,0.,0.));
#8024=CARTESIAN_POINT('',(86.5709088298366,-3.45978675425269,0.000812295043242979));
#8025=CARTESIAN_POINT('',(86.868373286472,-3.44956363082089,-0.00156881125221945));
#8026=CARTESIAN_POINT('',(84.65,-3.4544,-4.23041990297462E-16));
#8027=CARTESIAN_POINT('Ctrl Pts',(86.868373286472,-3.44956363082089,-0.00156881125221945));
#8028=CARTESIAN_POINT('Ctrl Pts',(86.8913616617206,-3.45151572191023,-0.474576012219106));
#8029=CARTESIAN_POINT('Ctrl Pts',(86.9143500369692,-3.3608767438491,-0.946867197435236));
#8030=CARTESIAN_POINT('Ctrl Pts',(86.9373384122178,-3.17403716751804,-1.37741099447087));
#8031=CARTESIAN_POINT('Ctrl Pts',(86.9931681812242,-2.7202769397939,-2.42303342214078));
#8032=CARTESIAN_POINT('Ctrl Pts',(87.0489979502306,-1.69911207658363,-3.22242389284734));
#8033=CARTESIAN_POINT('Ctrl Pts',(87.1048277192369,-0.575133802999295,-3.41189010624943));
#8034=CARTESIAN_POINT('Ctrl Pts',(87.1606574882433,0.548844470585059,-3.60135631965152));
#8035=CARTESIAN_POINT('Ctrl Pts',(87.2164872572496,1.77563615454348,-3.18089827574911));
#8036=CARTESIAN_POINT('Ctrl Pts',(87.272317026256,2.54709763079675,-2.34180841395378));
#8037=CARTESIAN_POINT('Ctrl Pts',(87.3281467952623,3.31855910705,-1.50271855215846));
#8038=CARTESIAN_POINT('Ctrl Pts',(87.3839765642687,3.6346903755981,-0.244996872470229));
#8039=CARTESIAN_POINT('Ctrl Pts',(87.4398063332751,3.35166371709586,0.859141033811245));
#8040=CARTESIAN_POINT('Ctrl Pts',(87.4956361022814,3.06863705859362,1.96327894009272));
#8041=CARTESIAN_POINT('Ctrl Pts',(87.5514658712878,2.18645247304104,2.91383307296744));
#8042=CARTESIAN_POINT('Ctrl Pts',(87.6072956402942,1.106470438205,3.27833740756711));
#8043=CARTESIAN_POINT('Ctrl Pts',(87.6631254093005,0.026488403368936,3.64284174216678));
#8044=CARTESIAN_POINT('Ctrl Pts',(87.7189551783069,-1.25129108075059,3.4212962784914));
#8045=CARTESIAN_POINT('Ctrl Pts',(87.7747849473132,-2.14552688370774,2.71449578739078));
#8046=CARTESIAN_POINT('Ctrl Pts',(87.8254255048106,-2.95664611994735,2.07339030646564));
#8047=CARTESIAN_POINT('Ctrl Pts',(87.876066062308,-3.45220667922921,1.03304363878092));
#8048=CARTESIAN_POINT('Ctrl Pts',(87.9267066198054,-3.45881529047273,-0.00181033228093454));
#8049=CARTESIAN_POINT('Ctrl Pts',(87.6292421631699,-3.45063882513586,0.00234158759808215));
#8050=CARTESIAN_POINT('Ctrl Pts',(87.6092538211845,-3.45322151305876,0.413298783665407));
#8051=CARTESIAN_POINT('Ctrl Pts',(87.5892654791991,-3.38530207254061,0.823430498208507));
#8052=CARTESIAN_POINT('Ctrl Pts',(87.5692771372136,-3.24307059694375,1.20592942853766));
#8053=CARTESIAN_POINT('Ctrl Pts',(87.5134473682073,-2.84580150710126,2.27429352502138));
#8054=CARTESIAN_POINT('Ctrl Pts',(87.457617599201,-1.86878706684323,3.12708045220674));
#8055=CARTESIAN_POINT('Ctrl Pts',(87.4017878301946,-0.756531735836134,3.37630455025122));
#8056=CARTESIAN_POINT('Ctrl Pts',(87.3459580611882,0.355723595170976,3.62552864829569));
#8057=CARTESIAN_POINT('Ctrl Pts',(87.2901282921818,1.60321981692717,3.27118991719926));
#8058=CARTESIAN_POINT('Ctrl Pts',(87.2342985231755,2.41839353309076,2.47449902050477));
#8059=CARTESIAN_POINT('Ctrl Pts',(87.1784687541691,3.23356724925433,1.67780812381029));
#8060=CARTESIAN_POINT('Ctrl Pts',(87.1226389851628,3.61641845982532,0.438765061517766));
#8061=CARTESIAN_POINT('Ctrl Pts',(87.0668092161565,3.39276440611025,-0.678912636504609));
#8062=CARTESIAN_POINT('Ctrl Pts',(87.0109794471501,3.16911035239517,-1.796590334527));
#8063=CARTESIAN_POINT('Ctrl Pts',(86.9551496781437,2.33895103439404,-2.79290266827921));
#8064=CARTESIAN_POINT('Ctrl Pts',(86.8993199091373,1.27997740925145,-3.2145653695609));
#8065=CARTESIAN_POINT('Ctrl Pts',(86.843490140131,0.221003784108877,-3.63622807084259));
#8066=CARTESIAN_POINT('Ctrl Pts',(86.7876603711246,-1.06678414817515,-3.48324113965374));
#8067=CARTESIAN_POINT('Ctrl Pts',(86.7318306021183,-1.99749179339816,-2.82520781867127));
#8068=CARTESIAN_POINT('Ctrl Pts',(86.6781900113577,-2.89170484144875,-2.19297708037795));
#8069=CARTESIAN_POINT('Ctrl Pts',(86.6245494205971,-3.4562919977347,-1.09453083635498));
#8070=CARTESIAN_POINT('Ctrl Pts',(86.5709088298366,-3.45978675425269,0.00081229504324298));
#8071=CARTESIAN_POINT('Origin',(84.65,0.,0.));
#8072=CARTESIAN_POINT('',(85.5125754965032,-3.45287610787495,-0.00301865808173374));
#8073=CARTESIAN_POINT('',(85.8100399531387,-3.45320716154862,0.00305860587857352));
#8074=CARTESIAN_POINT('',(84.65,-3.4544,-4.23041990297462E-16));
#8075=CARTESIAN_POINT('Ctrl Pts',(85.8100399531387,-3.45320716154862,0.00305860587857352));
#8076=CARTESIAN_POINT('Ctrl Pts',(85.8508274921269,-3.44594376666017,-0.833950371543459));
#8077=CARTESIAN_POINT('Ctrl Pts',(85.8916150311151,-3.13961127392647,-1.67572430432957));
#8078=CARTESIAN_POINT('Ctrl Pts',(85.9324025701033,-2.58649539295724,-2.29821986996156));
#8079=CARTESIAN_POINT('Ctrl Pts',(85.9882323391097,-1.82939328201139,-3.15028852864581));
#8080=CARTESIAN_POINT('Ctrl Pts',(86.0440621081161,-0.609918048706947,-3.5915174464072));
#8081=CARTESIAN_POINT('Ctrl Pts',(86.0998918771225,0.517115396018346,-3.42116422518358));
#8082=CARTESIAN_POINT('Ctrl Pts',(86.1557216461288,1.64414884074359,-3.25081100395996));
#8083=CARTESIAN_POINT('Ctrl Pts',(86.2115514151351,2.67874049688969,-2.46887564375138));
#8084=CARTESIAN_POINT('Ctrl Pts',(86.2673811841415,3.15019045855844,-1.43110903263256));
#8085=CARTESIAN_POINT('Ctrl Pts',(86.3232109531478,3.62164042022721,-0.393342421513706));
#8086=CARTESIAN_POINT('Ctrl Pts',(86.3790407221543,3.52994868741858,0.900255440515412));
#8087=CARTESIAN_POINT('Ctrl Pts',(86.4348704911606,2.91683151576663,1.86114666190112));
#8088=CARTESIAN_POINT('Ctrl Pts',(86.490700260167,2.3037143441147,2.82203788328681));
#8089=CARTESIAN_POINT('Ctrl Pts',(86.5465300291733,1.16917173361946,3.45022246402909));
#8090=CARTESIAN_POINT('Ctrl Pts',(86.6023597981796,0.0293774778981162,3.4599002806826));
#8091=CARTESIAN_POINT('Ctrl Pts',(86.658189567186,-1.11041677782324,3.4695780973361));
#8092=CARTESIAN_POINT('Ctrl Pts',(86.7140193361924,-2.25546267877071,2.8607491499008));
#8093=CARTESIAN_POINT('Ctrl Pts',(86.7698491051988,-2.88480783312544,1.91040748386653));
#8094=CARTESIAN_POINT('Ctrl Pts',(86.8026904989565,-3.25501484618601,1.35137696280011));
#8095=CARTESIAN_POINT('Ctrl Pts',(86.8355318927143,-3.44677485643284,0.67417340929306));
#8096=CARTESIAN_POINT('Ctrl Pts',(86.868373286472,-3.44956363082089,-0.00156881125221945));
#8097=CARTESIAN_POINT('Ctrl Pts',(86.5709088298366,-3.45978675425269,0.00081229504324298));
#8098=CARTESIAN_POINT('Ctrl Pts',(86.5687196515908,-3.45992938215508,0.0455154073866809));
#8099=CARTESIAN_POINT('Ctrl Pts',(86.566530473345,-3.45913744502121,0.0902133511329964));
#8100=CARTESIAN_POINT('Ctrl Pts',(86.5643412950992,-3.45739520842613,0.134874223357528));
#8101=CARTESIAN_POINT('Ctrl Pts',(86.5085115260929,-3.41296362006907,1.27384323362772));
#8102=CARTESIAN_POINT('Ctrl Pts',(86.4526817570865,-2.75047308519294,2.388701543392));
#8103=CARTESIAN_POINT('Ctrl Pts',(86.3968519880802,-1.77133163330598,2.97223096818263));
#8104=CARTESIAN_POINT('Ctrl Pts',(86.3410222190738,-0.792190181419031,3.55576039297326));
#8105=CARTESIAN_POINT('Ctrl Pts',(86.2851924500674,0.503602187478725,3.60796093279025));
#8106=CARTESIAN_POINT('Ctrl Pts',(86.229362681061,1.52650916456398,3.10508332478799));
#8107=CARTESIAN_POINT('Ctrl Pts',(86.1735329120547,2.54941614164925,2.60220571678573));
#8108=CARTESIAN_POINT('Ctrl Pts',(86.1177031430483,3.299437726922,1.54424996096417));
#8109=CARTESIAN_POINT('Ctrl Pts',(86.061873374042,3.43534258769914,0.412545741118299));
#8110=CARTESIAN_POINT('Ctrl Pts',(86.0060436050356,3.57124744847628,-0.719158478727583));
#8111=CARTESIAN_POINT('Ctrl Pts',(85.9502138360292,3.09303558475781,-1.92461116259779));
#8112=CARTESIAN_POINT('Ctrl Pts',(85.8943840670229,2.21827523026619,-2.65537712691846));
#8113=CARTESIAN_POINT('Ctrl Pts',(85.8385542980165,1.34351487577459,-3.38614309123912));
#8114=CARTESIAN_POINT('Ctrl Pts',(85.7827245290102,0.072206030509842,-3.64222233601026));
#8115=CARTESIAN_POINT('Ctrl Pts',(85.7268947600038,-1.0172540699822,-3.30710853170544));
#8116=CARTESIAN_POINT('Ctrl Pts',(85.6710649909975,-2.10671417047426,-2.97199472740061));
#8117=CARTESIAN_POINT('Ctrl Pts',(85.6152352219911,-3.01432552619362,-2.04568787401981));
#8118=CARTESIAN_POINT('Ctrl Pts',(85.5594054529847,-3.32715944475099,-0.949622405263555));
#8119=CARTESIAN_POINT('Ctrl Pts',(85.5437954674909,-3.41462770796557,-0.643162852016612));
#8120=CARTESIAN_POINT('Ctrl Pts',(85.528185481997,-3.4555986618466,-0.323432252563192));
#8121=CARTESIAN_POINT('Ctrl Pts',(85.5125754965032,-3.45287610787495,-0.00301865808173374));
#8122=CARTESIAN_POINT('Origin',(84.65,0.,0.));
#8123=CARTESIAN_POINT('',(84.4542421631699,-3.44973260108164,0.00172992572337771));
#8124=CARTESIAN_POINT('',(84.7517066198054,-3.45965414368361,-0.0010147492130462));
#8125=CARTESIAN_POINT('',(84.65,-3.4544,-4.23041990297462E-16));
#8126=CARTESIAN_POINT('Ctrl Pts',(84.7517066198054,-3.45965414368361,-0.0010147492130462));
#8127=CARTESIAN_POINT('Ctrl Pts',(84.7544635535269,-3.45987358617366,-0.0573172245063646));
#8128=CARTESIAN_POINT('Ctrl Pts',(84.7572204872483,-3.45861734950704,-0.11360970225368));
#8129=CARTESIAN_POINT('Ctrl Pts',(84.7599774209698,-3.45585465379575,-0.169828149355248));
#8130=CARTESIAN_POINT('Ctrl Pts',(84.8158071899762,-3.39990820060586,-1.30828965502245));
#8131=CARTESIAN_POINT('Ctrl Pts',(84.8716369589825,-2.72617819711704,-2.41639194493554));
#8132=CARTESIAN_POINT('Ctrl Pts',(84.9274667279889,-1.74118620413938,-2.98999056704028));
#8133=CARTESIAN_POINT('Ctrl Pts',(84.9832964969953,-0.756194211161706,-3.56358918914502));
#8134=CARTESIAN_POINT('Ctrl Pts',(85.0391262660017,0.540059771304828,-3.60268414344138));
#8135=CARTESIAN_POINT('Ctrl Pts',(85.094956035008,1.55782941779685,-3.08948871069662));
#8136=CARTESIAN_POINT('Ctrl Pts',(85.1507858040143,2.57559906428888,-2.57629327795187));
#8137=CARTESIAN_POINT('Ctrl Pts',(85.2066155730207,3.31488437480642,-1.510807458166));
#8138=CARTESIAN_POINT('Ctrl Pts',(85.262445342027,3.43933861387626,-0.377786828217834));
#8139=CARTESIAN_POINT('Ctrl Pts',(85.3182751110334,3.56379285294609,0.7552338017303));
#8140=CARTESIAN_POINT('Ctrl Pts',(85.3741048800397,3.07341602056828,1.95578924184072));
#8141=CARTESIAN_POINT('Ctrl Pts',(85.4299346490461,2.1913109491344,2.67767236843473));
#8142=CARTESIAN_POINT('Ctrl Pts',(85.4857644180525,1.30920587770051,3.39955549502874));
#8143=CARTESIAN_POINT('Ctrl Pts',(85.5415941870588,0.0353725672105228,3.64276630810633));
#8144=CARTESIAN_POINT('Ctrl Pts',(85.5974239560652,-1.05064321100081,3.2966531257706));
#8145=CARTESIAN_POINT('Ctrl Pts',(85.6532537250716,-2.13665898921217,2.95053994343486));
#8146=CARTESIAN_POINT('Ctrl Pts',(85.7090834940779,-3.03485723514488,2.01510276568579));
#8147=CARTESIAN_POINT('Ctrl Pts',(85.7649132630843,-3.3365918638176,0.915929977007713));
#8148=CARTESIAN_POINT('Ctrl Pts',(85.7799554931024,-3.41788830780643,0.619779550250641));
#8149=CARTESIAN_POINT('Ctrl Pts',(85.7949977231206,-3.45588586341039,0.311743117814283));
#8150=CARTESIAN_POINT('Ctrl Pts',(85.8100399531387,-3.45320716154862,0.00305860587857352));
#8151=CARTESIAN_POINT('Ctrl Pts',(85.5125754965032,-3.45287610787495,-0.00301865808173374));
#8152=CARTESIAN_POINT('Ctrl Pts',(85.4723557129907,-3.44586133317295,0.822540430977856));
#8153=CARTESIAN_POINT('Ctrl Pts',(85.4321359294782,-3.14878420194866,1.65263362949813));
#8154=CARTESIAN_POINT('Ctrl Pts',(85.3919161459656,-2.60960248063633,2.2719479695695));
#8155=CARTESIAN_POINT('Ctrl Pts',(85.3360863769593,-1.86115511656889,3.13162879151465));
#8156=CARTESIAN_POINT('Ctrl Pts',(85.2802566079529,-0.6462039070386,3.58516635127327));
#8157=CARTESIAN_POINT('Ctrl Pts',(85.2244268389466,0.482494495994766,3.42621828620259));
#8158=CARTESIAN_POINT('Ctrl Pts',(85.1685970699402,1.61119289902813,3.26727022113191));
#8159=CARTESIAN_POINT('Ctrl Pts',(85.1127673009339,2.65363849556458,2.49583653123193));
#8160=CARTESIAN_POINT('Ctrl Pts',(85.0569375319275,3.13555813515021,1.46289024347954));
#8161=CARTESIAN_POINT('Ctrl Pts',(85.0011077629212,3.61747777473585,0.42994395572713));
#8162=CARTESIAN_POINT('Ctrl Pts',(84.9452779939148,3.53887145737065,-0.864514929877678));
#8163=CARTESIAN_POINT('Ctrl Pts',(84.8894482249084,2.9355020716948,-1.83155678875917));
#8164=CARTESIAN_POINT('Ctrl Pts',(84.833618455902,2.33213268601896,-2.79859864764063));
#8165=CARTESIAN_POINT('Ctrl Pts',(84.7777886868957,1.2040002320325,-3.43822347979879));
#8166=CARTESIAN_POINT('Ctrl Pts',(84.7219589178894,0.0643621256227443,-3.45942628193745));
#8167=CARTESIAN_POINT('Ctrl Pts',(84.666129148883,-1.07527598078704,-3.48062908407612));
#8168=CARTESIAN_POINT('Ctrl Pts',(84.6102993798766,-2.22641973962013,-2.88340985619525));
#8169=CARTESIAN_POINT('Ctrl Pts',(84.5544696108703,-2.86534246533909,-1.93948066236783));
#8170=CARTESIAN_POINT('Ctrl Pts',(84.5210604616368,-3.24768086780961,-1.37462302702994));
#8171=CARTESIAN_POINT('Ctrl Pts',(84.4876513124034,-3.44659509347488,-0.685610025194725));
#8172=CARTESIAN_POINT('Ctrl Pts',(84.4542421631699,-3.44973260108164,0.00172992572337771));
#8173=CARTESIAN_POINT('Origin',(84.65,0.,0.));
#8174=CARTESIAN_POINT('',(83.3959088298365,-3.45904630125211,0.00163698504970649));
#8175=CARTESIAN_POINT('',(83.6933732864721,-3.45040227751753,-0.00221153198392862));
#8176=CARTESIAN_POINT('',(84.65,-3.4544,-4.23041990297462E-16));
#8177=CARTESIAN_POINT('Ctrl Pts',(83.6933732864721,-3.45040227751753,-0.00221153198392862));
#8178=CARTESIAN_POINT('Ctrl Pts',(83.7139293839331,-3.45289985741792,-0.424914548013618));
#8179=CARTESIAN_POINT('Ctrl Pts',(83.7344854813943,-3.38095223892544,-0.84679701239954));
#8180=CARTESIAN_POINT('Ctrl Pts',(83.7550415788554,-3.23071059867279,-1.23866138072456));
#8181=CARTESIAN_POINT('Ctrl Pts',(83.8108713478617,-2.82265862838445,-2.30295372545619));
#8182=CARTESIAN_POINT('Ctrl Pts',(83.866701116868,-1.8370708345208,-3.1458175953063));
#8183=CARTESIAN_POINT('Ctrl Pts',(83.9225308858744,-0.722352226990953,-3.38378194460523));
#8184=CARTESIAN_POINT('Ctrl Pts',(83.9783606548808,0.392366380538912,-3.62174629390416));
#8185=CARTESIAN_POINT('Ctrl Pts',(84.0341904238871,1.636215801735,-3.25481112265189));
#8186=CARTESIAN_POINT('Ctrl Pts',(84.0900201928935,2.44329179599138,-2.44991799620239));
#8187=CARTESIAN_POINT('Ctrl Pts',(84.1458499618999,3.25036779024777,-1.6450248697529));
#8188=CARTESIAN_POINT('Ctrl Pts',(84.2016797309063,3.62067035756447,-0.402173788106215));
#8189=CARTESIAN_POINT('Ctrl Pts',(84.2575094999126,3.38572589528446,0.713185214706118));
#8190=CARTESIAN_POINT('Ctrl Pts',(84.313339268919,3.15078143300445,1.82854421751844));
#8191=CARTESIAN_POINT('Ctrl Pts',(84.3691690379253,2.31058994112772,2.8164111414964));
#8192=CARTESIAN_POINT('Ctrl Pts',(84.4249988069317,1.24740663485295,3.22734405909875));
#8193=CARTESIAN_POINT('Ctrl Pts',(84.480828575938,0.184223328578151,3.6382769767011));
#8194=CARTESIAN_POINT('Ctrl Pts',(84.5366583449444,-1.10195179209471,3.47227588792783));
#8195=CARTESIAN_POINT('Ctrl Pts',(84.5924881139508,-2.02595790098566,2.80486498283053));
#8196=CARTESIAN_POINT('Ctrl Pts',(84.6455609492356,-2.90433559969705,2.17041154223815));
#8197=CARTESIAN_POINT('Ctrl Pts',(84.6986337845205,-3.45542972760911,1.08284590876941));
#8198=CARTESIAN_POINT('Ctrl Pts',(84.7517066198054,-3.45965414368361,-0.0010147492130462));
#8199=CARTESIAN_POINT('Ctrl Pts',(84.4542421631699,-3.44973260108164,0.00172992572337771));
#8200=CARTESIAN_POINT('Ctrl Pts',(84.431821543397,-3.45183815799343,0.462998411986782));
#8201=CARTESIAN_POINT('Ctrl Pts',(84.4094009236241,-3.36577278153509,0.923513415086305));
#8202=CARTESIAN_POINT('Ctrl Pts',(84.3869803038512,-3.18780308562104,1.34524502254394));
#8203=CARTESIAN_POINT('Ctrl Pts',(84.3311505348448,-2.74463928757921,2.39540235385431));
#8204=CARTESIAN_POINT('Ctrl Pts',(84.2753207658384,-1.73160999889071,3.20507785670111));
#8205=CARTESIAN_POINT('Ctrl Pts',(84.2194909968321,-0.609605067279678,3.40589993178326));
#8206=CARTESIAN_POINT('Ctrl Pts',(84.1636612278257,0.512399864331356,3.60672200686541));
#8207=CARTESIAN_POINT('Ctrl Pts',(84.1078314588194,1.74338043886494,3.19869065418292));
#8208=CARTESIAN_POINT('Ctrl Pts',(84.052001689813,2.52328725213983,2.36744464065433));
#8209=CARTESIAN_POINT('Ctrl Pts',(83.9961719208067,3.30319406541474,1.53619862712572));
#8210=CARTESIAN_POINT('Ctrl Pts',(83.9403421518003,3.63202711743095,0.281737952751017));
#8211=CARTESIAN_POINT('Ctrl Pts',(83.8845123827939,3.36017985982636,-0.825205424722592));
#8212=CARTESIAN_POINT('Ctrl Pts',(83.8286826137876,3.08833260222177,-1.93214880219619));
#8213=CARTESIAN_POINT('Ctrl Pts',(83.7728528447812,2.21580503499638,-2.89157488276869));
#8214=CARTESIAN_POINT('Ctrl Pts',(83.7170230757749,1.1395640593878,-3.26698124235905));
#8215=CARTESIAN_POINT('Ctrl Pts',(83.6611933067685,0.0633230837792188,-3.64238760194941));
#8216=CARTESIAN_POINT('Ctrl Pts',(83.6053635377622,-1.21663130021256,-3.43377424055763));
#8217=CARTESIAN_POINT('Ctrl Pts',(83.5495337687558,-2.11796846531068,-2.73605231370378));
#8218=CARTESIAN_POINT('Ctrl Pts',(83.4983254557827,-2.94469507489686,-2.09608615524738));
#8219=CARTESIAN_POINT('Ctrl Pts',(83.4471171428096,-3.45289220190666,-1.04463448977794));
#8220=CARTESIAN_POINT('Ctrl Pts',(83.3959088298365,-3.45904630125211,0.00163698504970649));
#8221=CARTESIAN_POINT('Origin',(84.65,0.,0.));
#8222=CARTESIAN_POINT('',(82.3375754965033,-3.45433093919597,-0.00310444462076481));
#8223=CARTESIAN_POINT('',(82.6350399531387,-3.4518452061196,0.00280651627479178));
#8224=CARTESIAN_POINT('',(84.65,-3.4544,-4.23041990297462E-16));
#8225=CARTESIAN_POINT('Ctrl Pts',(82.6350399531387,-3.4518452061196,0.00280651627479178));
#8226=CARTESIAN_POINT('Ctrl Pts',(82.6733952143394,-3.44576312325575,-0.785076990999158));
#8227=CARTESIAN_POINT('Ctrl Pts',(82.7117504755402,-3.17789065414655,-1.57670048768815));
#8228=CARTESIAN_POINT('Ctrl Pts',(82.7501057367409,-2.68359731851267,-2.18405091986124));
#8229=CARTESIAN_POINT('Ctrl Pts',(82.8059355057472,-1.9641058619064,-3.06810784641131));
#8230=CARTESIAN_POINT('Ctrl Pts',(82.8617652747536,-0.764882922038081,-3.56173436819202));
#8231=CARTESIAN_POINT('Ctrl Pts',(82.9175950437599,0.368470614410377,-3.44034916756878));
#8232=CARTESIAN_POINT('Ctrl Pts',(82.9734248127663,1.50182415085883,-3.31896396694554));
#8233=CARTESIAN_POINT('Ctrl Pts',(83.0292545817727,2.56930828388742,-2.58256704391836));
#8234=CARTESIAN_POINT('Ctrl Pts',(83.085084350779,3.0852582799953,-1.56619102736403));
#8235=CARTESIAN_POINT('Ctrl Pts',(83.1409141197854,3.60120827610318,-0.549815010809704));
#8236=CARTESIAN_POINT('Ctrl Pts',(83.1967438887917,3.56562413529035,0.746540099271768));
#8237=CARTESIAN_POINT('Ctrl Pts',(83.2525736577981,2.9946952900083,1.73308196819345));
#8238=CARTESIAN_POINT('Ctrl Pts',(83.3084034268044,2.42376644472625,2.71962383711512));
#8239=CARTESIAN_POINT('Ctrl Pts',(83.3642331958109,1.31749289497499,3.39635246487701));
#8240=CARTESIAN_POINT('Ctrl Pts',(83.4200629648172,0.179187085497533,3.45538203052369));
#8241=CARTESIAN_POINT('Ctrl Pts',(83.4758927338236,-0.959118723979919,3.51441159617038));
#8242=CARTESIAN_POINT('Ctrl Pts',(83.5317225028299,-2.12945679318357,2.95574209970188));
#8243=CARTESIAN_POINT('Ctrl Pts',(83.5875522718362,-2.79936775442887,2.03354694166105));
#8244=CARTESIAN_POINT('Ctrl Pts',(83.6228259433815,-3.22262258123717,1.45089704565928));
#8245=CARTESIAN_POINT('Ctrl Pts',(83.6580996149268,-3.44611650230016,0.723134676207329));
#8246=CARTESIAN_POINT('Ctrl Pts',(83.6933732864721,-3.45040227751753,-0.00221153198392862));
#8247=CARTESIAN_POINT('Ctrl Pts',(83.3959088298365,-3.45904630125211,0.00163698504970649));
#8248=CARTESIAN_POINT('Ctrl Pts',(83.3912873738032,-3.45960169739579,0.096061060733295));
#8249=CARTESIAN_POINT('Ctrl Pts',(83.38666591777,-3.45606808841924,0.190442945160575));
#8250=CARTESIAN_POINT('Ctrl Pts',(83.3820444617367,-3.44831058325344,0.284476369487177));
#8251=CARTESIAN_POINT('Ctrl Pts',(83.3262146927303,-3.35459558989358,1.42045263350827));
#8252=CARTESIAN_POINT('Ctrl Pts',(83.2703849237241,-2.64444565696942,2.50557466923451));
#8253=CARTESIAN_POINT('Ctrl Pts',(83.2145551547177,-1.6409520298194,3.04615316739094));
#8254=CARTESIAN_POINT('Ctrl Pts',(83.1587253857113,-0.637458402669365,3.58673166554739));
#8255=CARTESIAN_POINT('Ctrl Pts',(83.1028956167049,0.659378918706555,3.58276662613398));
#8256=CARTESIAN_POINT('Ctrl Pts',(83.0470658476985,1.65954821179859,3.03606199147685));
#8257=CARTESIAN_POINT('Ctrl Pts',(82.9912360786921,2.65971750489062,2.48935735681972));
#8258=CARTESIAN_POINT('Ctrl Pts',(82.9354063096858,3.36321876969879,1.39991312691889));
#8259=CARTESIAN_POINT('Ctrl Pts',(82.8795765406795,3.44998565233621,0.263385045225713));
#8260=CARTESIAN_POINT('Ctrl Pts',(82.8237467716731,3.53675253497364,-0.873143036467469));
#8261=CARTESIAN_POINT('Ctrl Pts',(82.7679170026668,3.0067850354403,-2.05675496995299));
#8262=CARTESIAN_POINT('Ctrl Pts',(82.7120872336604,2.10119823588243,-2.7489522834889));
#8263=CARTESIAN_POINT('Ctrl Pts',(82.656257464654,1.19561143632454,-3.44114959702482));
#8264=CARTESIAN_POINT('Ctrl Pts',(82.6004276956476,-0.0855946632578827,
-3.64193229061111));
#8265=CARTESIAN_POINT('Ctrl Pts',(82.5445979266412,-1.15951995253908,-3.25995186514127));
#8266=CARTESIAN_POINT('Ctrl Pts',(82.4887681576349,-2.23344524182026,-2.87797143967144));
#8267=CARTESIAN_POINT('Ctrl Pts',(82.4329383886286,-3.10008972080022,-1.91322789514549));
#8268=CARTESIAN_POINT('Ctrl Pts',(82.3771086196223,-3.36516306993141,-0.804642899766173));
#8269=CARTESIAN_POINT('Ctrl Pts',(82.3639309119159,-3.42772931689531,-0.542979466498652));
#8270=CARTESIAN_POINT('Ctrl Pts',(82.3507532042096,-3.45678088484327,-0.273302350699935));
#8271=CARTESIAN_POINT('Ctrl Pts',(82.3375754965033,-3.45433093919597,-0.00310444462076481));
#8272=CARTESIAN_POINT('Origin',(84.65,0.,0.));
#8273=CARTESIAN_POINT('',(81.2792421631699,-3.44913158907647,0.00100292261883378));
#8274=CARTESIAN_POINT('',(81.5767066198053,-3.46001944289485,-0.000122141770493717));
#8275=CARTESIAN_POINT('',(84.65,-3.4544,-4.23041990297462E-16));
#8276=CARTESIAN_POINT('Ctrl Pts',(81.5767066198053,-3.46001944289485,-0.000122141770493717));
#8277=CARTESIAN_POINT('Ctrl Pts',(81.5770312757393,-3.46002289260932,-0.00675043203261977));
#8278=CARTESIAN_POINT('Ctrl Pts',(81.5773559316733,-3.4600054815873,-0.013378703645769));
#8279=CARTESIAN_POINT('Ctrl Pts',(81.5776805876073,-3.45996715508333,-0.0200068543175971));
#8280=CARTESIAN_POINT('Ctrl Pts',(81.6335103566137,-3.45337630107705,-1.15982314045938));
#8281=CARTESIAN_POINT('Ctrl Pts',(81.68934012562,-2.82826672822439,-2.29606291464425));
#8282=CARTESIAN_POINT('Ctrl Pts',(81.7451698946264,-1.86903954818118,-2.91178023824083));
#8283=CARTESIAN_POINT('Ctrl Pts',(81.8009996636328,-0.909812368137995,-3.52749756183741));
#8284=CARTESIAN_POINT('Ctrl Pts',(81.8568294326391,0.383532419095744,-3.6226924348457));
#8285=CARTESIAN_POINT('Ctrl Pts',(81.9126592016455,1.42257206138549,-3.15405480590312));
#8286=CARTESIAN_POINT('Ctrl Pts',(81.9684889706519,2.46161170367527,-2.68541717696053));
#8287=CARTESIAN_POINT('Ctrl Pts',(82.0243187396582,3.24634620102107,-1.65294704606706));
#8288=CARTESIAN_POINT('Ctrl Pts',(82.0801485086645,3.4197511642724,-0.526379105714418));
#8289=CARTESIAN_POINT('Ctrl Pts',(82.1359782776709,3.59315612752373,0.600188834638211));
#8290=CARTESIAN_POINT('Ctrl Pts',(82.1918080466773,3.15523155668061,1.82085458444999));
#8291=CARTESIAN_POINT('Ctrl Pts',(82.2476378156836,2.30521649746879,2.58026159299263));
#8292=CARTESIAN_POINT('Ctrl Pts',(82.30346758469,1.45520143825698,3.33966860153526));
#8293=CARTESIAN_POINT('Ctrl Pts',(82.3592973536963,0.193095890676444,3.63781686880876));
#8294=CARTESIAN_POINT('Ctrl Pts',(82.4151271227027,-0.906890060597697,3.33906025798641));
#8295=CARTESIAN_POINT('Ctrl Pts',(82.4709568917091,-2.00687601187186,3.04030364716405));
#8296=CARTESIAN_POINT('Ctrl Pts',(82.5267866607154,-2.94474236683964,2.14464215824585));
#8297=CARTESIAN_POINT('Ctrl Pts',(82.5826164297218,-3.29379555765141,1.05956774812703));
#8298=CARTESIAN_POINT('Ctrl Pts',(82.6000909375274,-3.40304789410166,0.719943537123092));
#8299=CARTESIAN_POINT('Ctrl Pts',(82.617565445333,-3.45461617941379,0.361763177415482));
#8300=CARTESIAN_POINT('Ctrl Pts',(82.6350399531387,-3.4518452061196,0.00280651627479178));
#8301=CARTESIAN_POINT('Ctrl Pts',(82.3375754965033,-3.45433093919597,-0.00310444462076481));
#8302=CARTESIAN_POINT('Ctrl Pts',(82.2949234352032,-3.44640124199378,0.871440499769488));
#8303=CARTESIAN_POINT('Ctrl Pts',(82.2522713739032,-3.10845802640836,1.75144130367814));
#8304=CARTESIAN_POINT('Ctrl Pts',(82.2096193126031,-2.50876343656488,2.38282997772174));
#8305=CARTESIAN_POINT('Ctrl Pts',(82.1537895435968,-1.72378823478477,3.20929141359766));
#8306=CARTESIAN_POINT('Ctrl Pts',(82.0979597745904,-0.490335611942143,3.60978783911679));
#8307=CARTESIAN_POINT('Ctrl Pts',(82.0421300055841,0.630420339698764,3.40210859301528));
#8308=CARTESIAN_POINT('Ctrl Pts',(81.9863002365777,1.75117629133966,3.19442934691377));
#8309=CARTESIAN_POINT('Ctrl Pts',(81.9304704675714,2.75923557177884,2.37857442919163));
#8310=CARTESIAN_POINT('Ctrl Pts',(81.874640698565,3.19596949826618,1.32572683820102));
#8311=CARTESIAN_POINT('Ctrl Pts',(81.8188109295586,3.63270342475352,0.272879247210409));
#8312=CARTESIAN_POINT('Ctrl Pts',(81.7629811605522,3.49811199728901,-1.01696101704867));
#8313=CARTESIAN_POINT('Ctrl Pts',(81.7071513915459,2.85342920308481,-1.9569656272804));
#8314=CARTESIAN_POINT('Ctrl Pts',(81.6513216225396,2.20874640888062,-2.89697023751212));
#8315=CARTESIAN_POINT('Ctrl Pts',(81.5954918535332,1.05397224793672,-3.4871391937165));
#8316=CARTESIAN_POINT('Ctrl Pts',(81.5396620845269,-0.0855148991452379,
-3.45896803763762));
#8317=CARTESIAN_POINT('Ctrl Pts',(81.4838323155205,-1.22500204622719,-3.43079688155875));
#8318=CARTESIAN_POINT('Ctrl Pts',(81.4280025465141,-2.34920217944721,-2.78428561319665));
#8319=CARTESIAN_POINT('Ctrl Pts',(81.3721727775078,-2.94664693950248,-1.81357230274801));
#8320=CARTESIAN_POINT('Ctrl Pts',(81.3411959060618,-3.27813621229857,-1.27497681930224));
#8321=CARTESIAN_POINT('Ctrl Pts',(81.3102190346159,-3.44746224273321,-0.636574751997453));
#8322=CARTESIAN_POINT('Ctrl Pts',(81.2792421631699,-3.44913158907647,0.00100292261883378));
#8323=CARTESIAN_POINT('Origin',(84.65,0.,0.));
#8324=CARTESIAN_POINT('',(80.2209088298365,-3.45793510972046,0.00231429949518289));
#8325=CARTESIAN_POINT('',(80.5183732864721,-3.45151093143175,-0.00270500195080525));
#8326=CARTESIAN_POINT('',(84.65,-3.4544,-4.23041990297462E-16));
#8327=CARTESIAN_POINT('Ctrl Pts',(80.5183732864721,-3.45151093143175,-0.00270500195080525));
#8328=CARTESIAN_POINT('Ctrl Pts',(80.5364971061457,-3.45426214331332,-0.375090745122094));
#8329=CARTESIAN_POINT('Ctrl Pts',(80.5546209258193,-3.39869986199205,-0.746677677909009));
#8330=CARTESIAN_POINT('Ctrl Pts',(80.5727447454929,-3.28132205985502,-1.09758759467381));
#8331=CARTESIAN_POINT('Ctrl Pts',(80.6285745144992,-2.91974399861838,-2.17855286291426));
#8332=CARTESIAN_POINT('Ctrl Pts',(80.6844042835056,-1.97158258973338,-3.06330861746674));
#8333=CARTESIAN_POINT('Ctrl Pts',(80.7402340525119,-0.868215259536808,-3.34932459633046));
#8334=CARTESIAN_POINT('Ctrl Pts',(80.7960638215183,0.235152070659761,-3.63534057519418));
#8335=CARTESIAN_POINT('Ctrl Pts',(80.8518935905247,1.4937253221679,-3.32261677836914));
#8336=CARTESIAN_POINT('Ctrl Pts',(80.907723359531,2.33490147085537,-2.5534306549958));
#8337=CARTESIAN_POINT('Ctrl Pts',(80.9635531285374,3.17607761954284,-1.78424453162245));
#8338=CARTESIAN_POINT('Ctrl Pts',(81.0193828975437,3.59985666540964,-0.558596081700797));
#8339=CARTESIAN_POINT('Ctrl Pts',(81.0752126665501,3.41343523929463,0.565891204752768));
#8340=CARTESIAN_POINT('Ctrl Pts',(81.1310424355564,3.22701381317962,1.69037849120633));
#8341=CARTESIAN_POINT('Ctrl Pts',(81.1868722045628,2.4303919150828,2.7137046141918));
#8342=CARTESIAN_POINT('Ctrl Pts',(81.2427019735692,1.3860022499685,3.17029505749191));
#8343=CARTESIAN_POINT('Ctrl Pts',(81.2985317425755,0.341612584854186,3.62688550079202));
#8344=CARTESIAN_POINT('Ctrl Pts',(81.3543615115819,-0.950544847277621,3.51674026440676));
#8345=CARTESIAN_POINT('Ctrl Pts',(81.4101912805883,-1.90258749576358,2.88997124716479));
#8346=CARTESIAN_POINT('Ctrl Pts',(81.4656963936607,-2.84909391687946,2.26684695717687));
#8347=CARTESIAN_POINT('Ctrl Pts',(81.521201506733,-3.45942965915134,1.13308985888859));
#8348=CARTESIAN_POINT('Ctrl Pts',(81.5767066198053,-3.46001944289485,-0.000122141770493717));
#8349=CARTESIAN_POINT('Ctrl Pts',(81.2792421631699,-3.44913158907647,0.00100292261883378));
#8350=CARTESIAN_POINT('Ctrl Pts',(81.2543892656095,-3.45047091392514,0.512534652402619));
#8351=CARTESIAN_POINT('Ctrl Pts',(81.2295363680491,-3.3438907635004,1.02353572618038));
#8352=CARTESIAN_POINT('Ctrl Pts',(81.2046834704887,-3.12655411418531,1.48203645516729));
#8353=CARTESIAN_POINT('Ctrl Pts',(81.1488537014823,-2.63832714192235,2.51201655009872));
#8354=CARTESIAN_POINT('Ctrl Pts',(81.093023932476,-1.59118381050591,3.27706138742638));
#8355=CARTESIAN_POINT('Ctrl Pts',(81.0371941634696,-0.461534561322807,3.42910462542053));
#8356=CARTESIAN_POINT('Ctrl Pts',(80.9813643944633,0.668114687860321,3.58114786341467));
#8357=CARTESIAN_POINT('Ctrl Pts',(80.9255346254569,1.88026985481012,3.12018950207527));
#8358=CARTESIAN_POINT('Ctrl Pts',(80.8697048564505,2.62344638073682,2.25594808689628));
#8359=CARTESIAN_POINT('Ctrl Pts',(80.8138750874442,3.36662290666352,1.39170667171732));
#8360=CARTESIAN_POINT('Ctrl Pts',(80.7580453184378,3.64082079156714,0.124182202698778));
#8361=CARTESIAN_POINT('Ctrl Pts',(80.7022155494315,3.32129041287442,-0.969949832064032));
#8362=CARTESIAN_POINT('Ctrl Pts',(80.6463857804251,3.0017600341817,-2.06408186682685));
#8363=CARTESIAN_POINT('Ctrl Pts',(80.5905560114187,2.08850139189263,-2.98482146733395));
#8364=CARTESIAN_POINT('Ctrl Pts',(80.5347262424124,0.997012479280798,-3.31326708847092));
#8365=CARTESIAN_POINT('Ctrl Pts',(80.478896473406,-0.0944764333310358,-3.64171270960789));
#8366=CARTESIAN_POINT('Ctrl Pts',(80.4230667043997,-1.36419561626563,-3.37786435137473));
#8367=CARTESIAN_POINT('Ctrl Pts',(80.3672369353933,-2.23447106995624,-2.64176299483581));
#8368=CARTESIAN_POINT('Ctrl Pts',(80.3184609002077,-2.99479279268316,-1.99866333123865));
#8369=CARTESIAN_POINT('Ctrl Pts',(80.2696848650221,-3.45022889886461,-0.995104519048995));
#8370=CARTESIAN_POINT('Ctrl Pts',(80.2209088298365,-3.45793510972046,0.00231429949518289));
#8371=CARTESIAN_POINT('Origin',(84.65,0.,0.));
#8372=CARTESIAN_POINT('',(79.1625754965032,-3.45582574002253,-0.002961649045852));
#8373=CARTESIAN_POINT('',(79.4600399531387,-3.45067402916032,0.00235956821323163));
#8374=CARTESIAN_POINT('',(84.65,-3.4544,-4.23041990297462E-16));
#8375=CARTESIAN_POINT('Ctrl Pts',(79.4600399531387,-3.45067402916032,0.00235956821323163));
#8376=CARTESIAN_POINT('Ctrl Pts',(79.4959629365519,-3.44599371542453,-0.736192453848879));
#8377=CARTESIAN_POINT('Ctrl Pts',(79.5318859199652,-3.21354307753759,-1.47743314832035));
#8378=CARTESIAN_POINT('Ctrl Pts',(79.5678089033784,-2.77566385451523,-2.06578390812058));
#8379=CARTESIAN_POINT('Ctrl Pts',(79.6236386723848,-2.09513307585447,-2.98017029514507));
#8380=CARTESIAN_POINT('Ctrl Pts',(79.6794684413911,-0.918412601109804,-3.52526820087666));
#8381=CARTESIAN_POINT('Ctrl Pts',(79.7352982103975,0.219134449978267,-3.4530787829694));
#8382=CARTESIAN_POINT('Ctrl Pts',(79.7911279794038,1.35668150106635,-3.38088936506215));
#8383=CARTESIAN_POINT('Ctrl Pts',(79.8469577484102,2.45505512849783,-2.69141262351603));
#8384=CARTESIAN_POINT('Ctrl Pts',(79.9027875174166,3.0145370520976,-1.69833428688242));
#8385=CARTESIAN_POINT('Ctrl Pts',(79.9586172864229,3.57401897569738,-0.705255950248812));
#8386=CARTESIAN_POINT('Ctrl Pts',(80.0144470554293,3.59460919546544,0.591423981472296));
#8387=CARTESIAN_POINT('Ctrl Pts',(80.0702768244356,3.06693994351031,1.60176539210869));
#8388=CARTESIAN_POINT('Ctrl Pts',(80.126106593442,2.53927069155519,2.61210680274506));
#8389=CARTESIAN_POINT('Ctrl Pts',(80.1819363624483,1.46334196787692,3.33610969229675));
#8390=CARTESIAN_POINT('Ctrl Pts',(80.2377661314547,0.328660473959983,3.4443802463351));
#8391=CARTESIAN_POINT('Ctrl Pts',(80.293595900461,-0.806021019956969,3.55265080037346));
#8392=CARTESIAN_POINT('Ctrl Pts',(80.3494256694675,-1.99945528411258,3.04518901889848));
#8393=CARTESIAN_POINT('Ctrl Pts',(80.4052554384738,-2.70867505939625,2.15287073719677));
#8394=CARTESIAN_POINT('Ctrl Pts',(80.4429613878066,-3.1876633373092,1.55022257086274));
#8395=CARTESIAN_POINT('Ctrl Pts',(80.4806673371393,-3.44578713492097,0.772030027260836));
#8396=CARTESIAN_POINT('Ctrl Pts',(80.5183732864721,-3.45151093143175,-0.00270500195080525));
#8397=CARTESIAN_POINT('Ctrl Pts',(80.2209088298365,-3.45793510972046,0.00231429949518289));
#8398=CARTESIAN_POINT('Ctrl Pts',(80.2138550960157,-3.45904954142728,0.14655576617193));
#8399=CARTESIAN_POINT('Ctrl Pts',(80.206801362195,-3.45080040796966,0.290668824557857));
#8400=CARTESIAN_POINT('Ctrl Pts',(80.1997476283742,-3.4327556926168,0.433544736072098));
#8401=CARTESIAN_POINT('Ctrl Pts',(80.1439178593678,-3.28993313714013,1.56439675559642));
#8402=CARTESIAN_POINT('Ctrl Pts',(80.0880880903615,-2.53345630174016,2.61774643980037));
#8403=CARTESIAN_POINT('Ctrl Pts',(80.0322583213552,-1.50749341271405,3.1143596924703));
#8404=CARTESIAN_POINT('Ctrl Pts',(79.9764285523488,-0.481530523687946,3.61097294514022));
#8405=CARTESIAN_POINT('Ctrl Pts',(79.9205987833424,0.813918418964297,3.55084976627612));
#8406=CARTESIAN_POINT('Ctrl Pts',(79.8647690143361,1.78947335231774,2.96134391865517));
#8407=CARTESIAN_POINT('Ctrl Pts',(79.8089392453297,2.76502828567118,2.37183807103423));
#8408=CARTESIAN_POINT('Ctrl Pts',(79.7531094763234,3.42068920972583,1.25294955465644));
#8409=CARTESIAN_POINT('Ctrl Pts',(79.697279707317,3.45815530848054,0.113730144726209));
#8410=CARTESIAN_POINT('Ctrl Pts',(79.6414499383106,3.49562140723526,-1.02548926520403));
#8411=CARTESIAN_POINT('Ctrl Pts',(79.5856201693043,2.91489268069002,-2.18503956868671));
#8412=CARTESIAN_POINT('Ctrl Pts',(79.5297904002979,1.98017864118596,-2.83736942130582));
#8413=CARTESIAN_POINT('Ctrl Pts',(79.4739606312915,1.0454646016819,-3.48969927392492));
#8414=CARTESIAN_POINT('Ctrl Pts',(79.4181308622852,-0.243234750780984,-3.63480867568044));
#8415=CARTESIAN_POINT('Ctrl Pts',(79.3623010932788,-1.29961016044813,-3.20667836130879));
#8416=CARTESIAN_POINT('Ctrl Pts',(79.3064713242725,-2.35598557011526,-2.77854804693713));
#8417=CARTESIAN_POINT('Ctrl Pts',(79.2506415552661,-3.18003703698667,-1.77717801643833));
#8418=CARTESIAN_POINT('Ctrl Pts',(79.1948117862598,-3.39685244416281,-0.658153596465372));
#8419=CARTESIAN_POINT('Ctrl Pts',(79.1840663563409,-3.43858241734022,-0.442777486259295));
#8420=CARTESIAN_POINT('Ctrl Pts',(79.1733209264221,-3.45781803868262,-0.223043006372249));
#8421=CARTESIAN_POINT('Ctrl Pts',(79.1625754965032,-3.45582574002253,-0.002961649045852));
#8422=CARTESIAN_POINT('Origin',(84.65,0.,0.));
#8423=CARTESIAN_POINT('',(78.1042421631699,-3.44886665199893,0.000209781305364476));
#8424=CARTESIAN_POINT('',(78.4017066198053,-3.45980363531856,0.000782824143658126));
#8425=CARTESIAN_POINT('',(84.65,-3.4544,-4.23041990297462E-16));
#8426=CARTESIAN_POINT('Ctrl Pts',(78.4017066198053,-3.45980363531856,0.000782824143658126));
#8427=CARTESIAN_POINT('Ctrl Pts',(78.4554287669582,-3.45641942945665,-1.09621141280894));
#8428=CARTESIAN_POINT('Ctrl Pts',(78.5091509141111,-2.88987735601417,-2.19621591060466));
#8429=CARTESIAN_POINT('Ctrl Pts',(78.5628730612639,-1.99338590411892,-2.82810636555822));
#8430=CARTESIAN_POINT('Ctrl Pts',(78.6187028302703,-1.06172339008944,-3.48478708304715));
#8431=CARTESIAN_POINT('Ctrl Pts',(78.6745325992766,0.226285422716833,-3.63590325801604));
#8432=CARTESIAN_POINT('Ctrl Pts',(78.730362368283,1.28464545005932,-3.21270276560162));
#8433=CARTESIAN_POINT('Ctrl Pts',(78.7861921372894,2.3430054774018,-2.7895022731872));
#8434=CARTESIAN_POINT('Ctrl Pts',(78.8420219062958,3.1717167192805,-1.79198511338946));
#8435=CARTESIAN_POINT('Ctrl Pts',(78.8978516753021,3.39374703706223,-0.673983707137805));
#8436=CARTESIAN_POINT('Ctrl Pts',(78.9536814443085,3.61577735484395,0.44401769911385));
#8437=CARTESIAN_POINT('Ctrl Pts',(79.0095112133148,3.23112674852871,1.68250335181942));
#8438=CARTESIAN_POINT('Ctrl Pts',(79.0653409823211,2.4147966340945,2.47800932264061));
#8439=CARTESIAN_POINT('Ctrl Pts',(79.1211707513275,1.59846651966029,3.2735152934618));
#8440=CARTESIAN_POINT('Ctrl Pts',(79.1770005203339,0.350456897107113,3.62604158239858));
#8441=CARTESIAN_POINT('Ctrl Pts',(79.2328302893402,-0.761435259650085,3.37520211756753));
#8442=CARTESIAN_POINT('Ctrl Pts',(79.2886600583466,-1.87332741640728,3.12436265273647));
#8443=CARTESIAN_POINT('Ctrl Pts',(79.3444898273529,-2.84910210736849,2.27015743413759));
#8444=CARTESIAN_POINT('Ctrl Pts',(79.4003195963593,-3.24481891156067,1.20121739067945));
#8445=CARTESIAN_POINT('Ctrl Pts',(79.4202263819524,-3.3859165681846,0.820073770783605));
#8446=CARTESIAN_POINT('Ctrl Pts',(79.4401331675456,-3.45326763339901,0.411629493916263));
#8447=CARTESIAN_POINT('Ctrl Pts',(79.4600399531387,-3.45067402916032,0.00235956821323163));
#8448=CARTESIAN_POINT('Ctrl Pts',(79.1625754965032,-3.45582574002253,-0.002961649045852));
#8449=CARTESIAN_POINT('Ctrl Pts',(79.1174911574157,-3.44746670096746,0.920428351678523));
#8450=CARTESIAN_POINT('Ctrl Pts',(79.0724068183282,-3.06541784343642,1.84992467687227));
#8451=CARTESIAN_POINT('Ctrl Pts',(79.0273224792407,-2.40321705390905,2.48924094437753));
#8452=CARTESIAN_POINT('Ctrl Pts',(78.9714927102343,-1.58318690899829,3.28093225580035));
#8453=CARTESIAN_POINT('Ctrl Pts',(78.915662941228,-0.333547271695907,3.62763606919886));
#8454=CARTESIAN_POINT('Ctrl Pts',(78.8598331722216,0.777163289075481,3.3716153242409));
#8455=CARTESIAN_POINT('Ctrl Pts',(78.8040034032152,1.88787384984687,3.11559457928293));
#8456=CARTESIAN_POINT('Ctrl Pts',(78.7481736342089,2.85965533408728,2.25684927596851));
#8457=CARTESIAN_POINT('Ctrl Pts',(78.6923438652025,3.25038407819797,1.18607589779917));
#8458=CARTESIAN_POINT('Ctrl Pts',(78.6365140961962,3.64111282230867,0.115302519629842));
#8459=CARTESIAN_POINT('Ctrl Pts',(78.5806843271898,3.45078882628966,-1.1674989333944));
#8460=CARTESIAN_POINT('Ctrl Pts',(78.5248545581834,2.76600227941643,-2.07870250373423));
#8461=CARTESIAN_POINT('Ctrl Pts',(78.4690247891771,2.0812157325432,-2.98990607407406));
#8462=CARTESIAN_POINT('Ctrl Pts',(78.4131950201707,0.901966634815757,-3.52951176172949));
#8463=CARTESIAN_POINT('Ctrl Pts',(78.3573652511644,-0.235231467171954,-3.45201951840901));
#8464=CARTESIAN_POINT('Ctrl Pts',(78.301535482158,-1.37242956915966,-3.37452727508854));
#8465=CARTESIAN_POINT('Ctrl Pts',(78.2457057131517,-2.46757667540763,-2.67993710079217));
#8466=CARTESIAN_POINT('Ctrl Pts',(78.1898759441453,-3.02242244917052,-1.68426105623825));
#8467=CARTESIAN_POINT('Ctrl Pts',(78.1613313504868,-3.30610349311992,-1.17519271128376));
#8468=CARTESIAN_POINT('Ctrl Pts',(78.1327867568284,-3.44854635896393,-0.587418619717722));
#8469=CARTESIAN_POINT('Ctrl Pts',(78.1042421631699,-3.44886665199893,0.000209781305364476));
#8470=CARTESIAN_POINT('Origin',(84.65,0.,0.));
#8471=CARTESIAN_POINT('',(77.0459088298365,-3.45658164681457,0.00280094662916092));
#8472=CARTESIAN_POINT('',(77.343373286472,-3.45282914603924,-0.00301189592616661));
#8473=CARTESIAN_POINT('',(84.65,-3.4544,-4.23041990297462E-16));
#8474=CARTESIAN_POINT('Ctrl Pts',(77.343373286472,-3.45282914603924,-0.00301189592616661));
#8475=CARTESIAN_POINT('Ctrl Pts',(77.3590648283581,-3.45555696923012,-0.325110759859066));
#8476=CARTESIAN_POINT('Ctrl Pts',(77.3747563702442,-3.41414927856796,-0.646521813152243));
#8477=CARTESIAN_POINT('Ctrl Pts',(77.3904479121303,-3.32577665812594,-0.954454511638704));
#8478=CARTESIAN_POINT('Ctrl Pts',(77.4462776811367,-3.01135102541417,-2.05006458939772));
#8479=CARTESIAN_POINT('Ctrl Pts',(77.5021074501431,-2.10239494861453,-2.97505177244844));
#8480=CARTESIAN_POINT('Ctrl Pts',(77.5579372191495,-1.01244917268523,-3.30858262931605));
#8481=CARTESIAN_POINT('Ctrl Pts',(77.6137669881558,0.0774966032440712,-3.64211348618366));
#8482=CARTESIAN_POINT('Ctrl Pts',(77.6695967571622,1.34843207830302,-3.38418801686816));
#8483=CARTESIAN_POINT('Ctrl Pts',(77.7254265261685,2.22213001584954,-2.65215220736641));
#8484=CARTESIAN_POINT('Ctrl Pts',(77.7812562951749,3.09582795339607,-1.92011639786466));
#8485=CARTESIAN_POINT('Ctrl Pts',(77.8370860641813,3.57228835343016,-0.713970248176632));
#8486=CARTESIAN_POINT('Ctrl Pts',(77.8929158331876,3.43473976591166,0.41753540250213));
#8487=CARTESIAN_POINT('Ctrl Pts',(77.948745602194,3.29719117839316,1.54904105318089));
#8488=CARTESIAN_POINT('Ctrl Pts',(78.0045753712003,2.54563360332207,2.60590620485039));
#8489=CARTESIAN_POINT('Ctrl Pts',(78.0604051402067,1.52199722376043,3.10729743581821));
#8490=CARTESIAN_POINT('Ctrl Pts',(78.116234909213,0.498360844198792,3.60868866678604));
#8491=CARTESIAN_POINT('Ctrl Pts',(78.1720646782194,-0.797354339853391,3.55460597705218));
#8492=CARTESIAN_POINT('Ctrl Pts',(78.2278944472258,-1.77564715267084,2.9696548962903));
#8493=CARTESIAN_POINT('Ctrl Pts',(78.2837242162321,-2.7539399654883,2.38470381552842));
#8494=CARTESIAN_POINT('Ctrl Pts',(78.3395539852385,-3.41481040707101,1.26888434373852));
#8495=CARTESIAN_POINT('Ctrl Pts',(78.3953837542448,-3.45758752023603,0.129851977839085));
#8496=CARTESIAN_POINT('Ctrl Pts',(78.3974913760983,-3.45920239309224,0.0868525252361583));
#8497=CARTESIAN_POINT('Ctrl Pts',(78.3995989979518,-3.45993640414128,0.0438199912992089));
#8498=CARTESIAN_POINT('Ctrl Pts',(78.4017066198053,-3.45980363531856,0.000782824143658126));
#8499=CARTESIAN_POINT('Ctrl Pts',(78.1042421631699,-3.44886665199893,0.000209781305364476));
#8500=CARTESIAN_POINT('Ctrl Pts',(78.076956987822,-3.4491728133592,0.561911382426732));
#8501=CARTESIAN_POINT('Ctrl Pts',(78.0496718124741,-3.3196209391107,1.12347986544209));
#8502=CARTESIAN_POINT('Ctrl Pts',(78.0223866371262,-3.0594386069859,1.61604710434839));
#8503=CARTESIAN_POINT('Ctrl Pts',(77.9665568681198,-2.52706454976058,2.62391730556962));
#8504=CARTESIAN_POINT('Ctrl Pts',(77.9107270991135,-1.44777199403211,3.34289579320058));
#8505=CARTESIAN_POINT('Ctrl Pts',(77.8548973301072,-0.312598052546025,3.44587499691791));
#8506=CARTESIAN_POINT('Ctrl Pts',(77.7990675611008,0.822575888940055,3.54885420063523));
#8507=CARTESIAN_POINT('Ctrl Pts',(77.7432377920944,2.01363121618376,3.03583412043895));
#8508=CARTESIAN_POINT('Ctrl Pts',(77.687408023088,2.7186829870306,2.14021875184474));
#8509=CARTESIAN_POINT('Ctrl Pts',(77.6315782540817,3.42373475787744,1.24460338325053));
#8510=CARTESIAN_POINT('Ctrl Pts',(77.5757484850753,3.64278297232741,-0.0336072737416136));
#8511=CARTESIAN_POINT('Ctrl Pts',(77.519918716069,3.27616903077557,-1.11287463115828));
#8512=CARTESIAN_POINT('Ctrl Pts',(77.4640889470626,2.90955508922373,-2.19214198857496));
#8513=CARTESIAN_POINT('Ctrl Pts',(77.4082591780563,1.95727899167008,-3.07246604641616));
#8514=CARTESIAN_POINT('Ctrl Pts',(77.3524294090499,0.852590156611448,-3.35333533965697));
#8515=CARTESIAN_POINT('Ctrl Pts',(77.2965996400435,-0.252098678447182,-3.63420463289779));
#8516=CARTESIAN_POINT('Ctrl Pts',(77.2407698710372,-1.50920025101079,-3.31561916153822));
#8517=CARTESIAN_POINT('Ctrl Pts',(77.1849401020308,-2.34678102618597,-2.5425182006909));
#8518=CARTESIAN_POINT('Ctrl Pts',(77.1385963446327,-3.04204881856385,-1.90077448561923));
#8519=CARTESIAN_POINT('Ctrl Pts',(77.0922525872346,-3.44824574888005,-0.945846811171742));
#8520=CARTESIAN_POINT('Ctrl Pts',(77.0459088298365,-3.45658164681457,0.00280094662916092));
#8521=CARTESIAN_POINT('Origin',(84.65,0.,0.));
#8522=CARTESIAN_POINT('',(75.9875754965032,-3.45725565822888,-0.00252520199929829));
#8523=CARTESIAN_POINT('',(76.2850399531387,-3.44974973462971,0.00177277111675968));
#8524=CARTESIAN_POINT('',(84.65,-3.4544,-4.23041990297462E-16));
#8525=CARTESIAN_POINT('',(75.342557724821,2.66903922910597,-2.19296806941949));
#8526=CARTESIAN_POINT('Ctrl Pts',(75.9875754965032,-3.45725565822888,-0.00252520199929829));
#8527=CARTESIAN_POINT('Ctrl Pts',(75.9400588796282,-3.44912275835016,0.969407753130569));
#8528=CARTESIAN_POINT('Ctrl Pts',(75.8925422627532,-3.01962093091058,1.94744243616048));
#8529=CARTESIAN_POINT('Ctrl Pts',(75.8450256458782,-2.29316705426671,2.59066122337652));
#8530=CARTESIAN_POINT('Ctrl Pts',(75.7891958768718,-1.4396182371553,3.34641276194424));
#8531=CARTESIAN_POINT('Ctrl Pts',(75.7333661078655,-0.176123125833669,3.63994645726298));
#8532=CARTESIAN_POINT('Ctrl Pts',(75.6775363388591,0.92247066266989,3.33539582878245));
#8533=CARTESIAN_POINT('Ctrl Pts',(75.6217065698528,2.02106445117345,3.03084520030191));
#8534=CARTESIAN_POINT('Ctrl Pts',(75.5658768008464,2.95475691685894,2.12821024802208));
#8535=CARTESIAN_POINT('Ctrl Pts',(75.5100470318401,3.29846760420812,1.04342284236128));
#8536=CARTESIAN_POINT('Ctrl Pts',(75.4542172628337,3.64217829155731,-0.0413645632995172));
#8537=CARTESIAN_POINT('Ctrl Pts',(75.3983874938273,3.3959072005702,-1.30830442234129));
#8538=CARTESIAN_POINT('Ctrl Pts',(75.342557724821,2.66903922910596,-2.1929680694195));
#8539=CARTESIAN_POINT('',(75.342557724821,-2.66725710276986,-2.19542711810056));
#8540=CARTESIAN_POINT('Origin',(75.342557724821,0.,0.));
#8541=CARTESIAN_POINT('Ctrl Pts',(75.342557724821,-2.66725710276986,-2.19542711810056));
#8542=CARTESIAN_POINT('Ctrl Pts',(75.3552305591811,-2.5042708137433,-2.39790962253998));
#8543=CARTESIAN_POINT('Ctrl Pts',(75.3679033935413,-2.31900993594976,-2.58145235087825));
#8544=CARTESIAN_POINT('Ctrl Pts',(75.3805762279015,-2.11423969877341,-2.73967296209481));
#8545=CARTESIAN_POINT('Ctrl Pts',(75.4364059969078,-1.21213092688924,-3.43670883625072));
#8546=CARTESIAN_POINT('Ctrl Pts',(75.4922357659142,0.0686184225984726,-3.64228925741259));
#8547=CARTESIAN_POINT('Ctrl Pts',(75.5480655349206,1.14443454333613,-3.26502848098788));
#8548=CARTESIAN_POINT('Ctrl Pts',(75.6038953039269,2.22025066407378,-2.88776770456317));
#8549=CARTESIAN_POINT('Ctrl Pts',(75.6597250729332,3.09113355606137,-1.92766573055188));
#8550=CARTESIAN_POINT('Ctrl Pts',(75.7155548419396,3.36131099418083,-0.820474311753891));
#8551=CARTESIAN_POINT('Ctrl Pts',(75.7713846109459,3.63148843230029,0.286717107044106));
#8552=CARTESIAN_POINT('Ctrl Pts',(75.8272143799524,3.3009604165516,1.54099797062881));
#8553=CARTESIAN_POINT('Ctrl Pts',(75.8830441489587,2.51987823294149,2.37118396395587));
#8554=CARTESIAN_POINT('Ctrl Pts',(75.9388739179651,1.73879604933139,3.20136995728294));
#8555=CARTESIAN_POINT('Ctrl Pts',(75.9947036869714,0.507159697859874,3.60746108035237));
#8556=CARTESIAN_POINT('Ctrl Pts',(76.0505334559777,-0.614568213469516,3.4049720476312));
#8557=CARTESIAN_POINT('Ctrl Pts',(76.1063632249841,-1.73629612479891,3.20248301491003));
#8558=CARTESIAN_POINT('Ctrl Pts',(76.1621929939905,-2.74811559598618,2.39141382639824));
#8559=CARTESIAN_POINT('Ctrl Pts',(76.2180227629968,-3.18974546299614,1.34063282447457));
#8560=CARTESIAN_POINT('Ctrl Pts',(76.2403618263775,-3.366454014106,0.920185743662626));
#8561=CARTESIAN_POINT('Ctrl Pts',(76.2627008897581,-3.45187375359347,0.461360189413245));
#8562=CARTESIAN_POINT('Ctrl Pts',(76.2850399531387,-3.44974973462971,0.00177277111675968));
#8563=CARTESIAN_POINT('Origin',(73.0447820522122,0.,0.));
#8564=CARTESIAN_POINT('',(93.5153333974298,-3.96228178397161,0.000254737798764393));
#8565=CARTESIAN_POINT('',(93.6822820522122,-3.96673102035433,0.00521690610871163));
#8566=CARTESIAN_POINT('',(73.0447820522122,-3.96875,-4.10839266763092E-13));
#8567=CARTESIAN_POINT('',(93.8044,-2.97061198327647,-2.63181325464293));
#8568=CARTESIAN_POINT('Ctrl Pts',(93.6822820522122,-3.96673102035433,0.00521690610871168));
#8569=CARTESIAN_POINT('Ctrl Pts',(93.7229880348082,-3.95801329736185,-0.951787959283503));
#8570=CARTESIAN_POINT('Ctrl Pts',(93.7636940174041,-3.60663188570075,-1.91391720316181));
#8571=CARTESIAN_POINT('Ctrl Pts',(93.8044,-2.97061198327643,-2.63181325464298));
#8572=CARTESIAN_POINT('',(93.8044000000001,0.57142891900023,-3.92761210585551));
#8573=CARTESIAN_POINT('Origin',(93.8044,0.,0.));
#8574=CARTESIAN_POINT('Ctrl Pts',(93.5153333974298,-3.96228178397161,0.00025473779876474));
#8575=CARTESIAN_POINT('Ctrl Pts',(93.5431863282533,-3.96226415926583,-0.658364510072053));
#8576=CARTESIAN_POINT('Ctrl Pts',(93.6268690280832,-3.49522148123942,-2.63729827531904));
#8577=CARTESIAN_POINT('Ctrl Pts',(93.7232245622734,-1.34167057967468,-4.04359863780956));
#8578=CARTESIAN_POINT('Ctrl Pts',(93.7917271656399,0.27639455735742,-3.97383332500728));
#8579=CARTESIAN_POINT('Ctrl Pts',(93.8044,0.57142891900023,-3.92761210585551));
#8580=CARTESIAN_POINT('Origin',(73.0447820522122,0.,0.));
#8581=CARTESIAN_POINT('',(92.4570000640964,-3.97078332034416,0.00332551191120287));
#8582=CARTESIAN_POINT('',(92.6239487188789,-3.97480878038019,-0.00116026438185279));
#8583=CARTESIAN_POINT('',(73.0447820522122,-3.96875,-4.10839266763092E-13));
#8584=CARTESIAN_POINT('Ctrl Pts',(92.6239487188789,-3.97480878038019,-0.00116026438185197));
#8585=CARTESIAN_POINT('Ctrl Pts',(92.626624096208,-3.97504728960825,-0.0639306450881609));
#8586=CARTESIAN_POINT('Ctrl Pts',(92.6851292425436,-3.94532727312447,-1.43635923310198));
#8587=CARTESIAN_POINT('Ctrl Pts',(92.7994641578856,-2.36394076440595,-4.0456605360623));
#8588=CARTESIAN_POINT('Ctrl Pts',(92.9669534649047,2.10367480928929,-4.18746581500559));
#8589=CARTESIAN_POINT('Ctrl Pts',(93.1344427719237,4.65703774727922,-0.51765171101067));
#8590=CARTESIAN_POINT('Ctrl Pts',(93.3019320789428,2.97298396264366,3.62053493698499));
#8591=CARTESIAN_POINT('Ctrl Pts',(93.4694213859619,-1.41651251429978,4.46956712243346));
#8592=CARTESIAN_POINT('Ctrl Pts',(93.596204710385,-3.76325080247511,2.025591834054));
#8593=CARTESIAN_POINT('Ctrl Pts',(93.6671582658018,-3.96996997866256,0.360779805095954));
#8594=CARTESIAN_POINT('Ctrl Pts',(93.6822820522122,-3.96673102035433,0.00521690610871168));
#8595=CARTESIAN_POINT('Ctrl Pts',(92.4570000640964,-3.97078332034416,0.0033255119112029));
#8596=CARTESIAN_POINT('Ctrl Pts',(92.5026521586596,-3.9611636135282,-1.07063415837227));
#8597=CARTESIAN_POINT('Ctrl Pts',(92.6041340222292,-2.95791654582123,-3.47380932989873));
#8598=CARTESIAN_POINT('Ctrl Pts',(92.761445654805,1.09859778933808,-4.55527773120639));
#8599=CARTESIAN_POINT('Ctrl Pts',(92.9289349618241,4.4179760167816,-1.56159205661129));
#8600=CARTESIAN_POINT('Ctrl Pts',(93.0964242688432,3.71721744660719,2.85269706473892));
#8601=CARTESIAN_POINT('Ctrl Pts',(93.2639135758623,-0.365701395163535,4.67189257704037));
#8602=CARTESIAN_POINT('Ctrl Pts',(93.4035499520579,-3.49259078967768,2.64337465166492));
#8603=CARTESIAN_POINT('Ctrl Pts',(93.487356559247,-3.96229948708317,0.661803938436363));
#8604=CARTESIAN_POINT('Ctrl Pts',(93.5153333974298,-3.96228178397161,0.00025473779876474));
#8605=CARTESIAN_POINT('Origin',(73.0447820522122,0.,0.));
#8606=CARTESIAN_POINT('',(91.3986667307631,-3.97246823586828,-0.00280997941530858));
#8607=CARTESIAN_POINT('',(91.5656153855456,-3.96419497404471,-0.00256333403586442));
#8608=CARTESIAN_POINT('',(73.0447820522122,-3.96875,-4.10839266763092E-13));
#8609=CARTESIAN_POINT('Ctrl Pts',(91.5656153855456,-3.96419497404471,-0.00256333403586429));
#8610=CARTESIAN_POINT('Ctrl Pts',(91.5860899266144,-3.96707960586625,-0.486267227833301));
#8611=CARTESIAN_POINT('Ctrl Pts',(91.6623942366896,-3.66153217022063,-2.28541151142624));
#8612=CARTESIAN_POINT('Ctrl Pts',(91.7945283157709,-0.984921998283766,-4.58115525704141));
#8613=CARTESIAN_POINT('Ctrl Pts',(91.9620176227903,3.30407582270753,-3.32268146160252));
#8614=CARTESIAN_POINT('Ctrl Pts',(92.1295069298092,4.58661448010922,0.959202947931876));
#8615=CARTESIAN_POINT('Ctrl Pts',(92.2969962368283,1.69568469472483,4.36824040377796));
#8616=CARTESIAN_POINT('Ctrl Pts',(92.4618101665183,-2.66736966883454,3.81163512773909));
#8617=CARTESIAN_POINT('Ctrl Pts',(92.5707943272017,-3.97007007949167,1.24596153985253));
#8618=CARTESIAN_POINT('Ctrl Pts',(92.6239487188789,-3.97480878038019,-0.00116026438185197));
#8619=CARTESIAN_POINT('Ctrl Pts',(91.3986667307631,-3.97246823586828,-0.00280997941530784));
#8620=CARTESIAN_POINT('Ctrl Pts',(91.4062882200596,-3.97390842000699,-0.181907740360926));
#8621=CARTESIAN_POINT('Ctrl Pts',(91.4697394783624,-3.88173674403366,-1.67146133766004));
#8622=CARTESIAN_POINT('Ctrl Pts',(91.5890205056715,-1.99881293045711,-4.2381396621777));
#8623=CARTESIAN_POINT('Ctrl Pts',(91.7565098126906,2.46387542085175,-3.98577567712814));
#8624=CARTESIAN_POINT('Ctrl Pts',(91.9239991197097,4.68462530132107,-0.10665579043167));
#8625=CARTESIAN_POINT('Ctrl Pts',(92.0914884267288,2.64272008949707,3.86950719504337));
#8626=CARTESIAN_POINT('Ctrl Pts',(92.2589777337479,-1.80385580473937,4.3247235657652));
#8627=CARTESIAN_POINT('Ctrl Pts',(92.3808149462037,-3.84445876308829,1.79327554700216));
#8628=CARTESIAN_POINT('Ctrl Pts',(92.4468223896532,-3.97292793704025,0.242753998025987));
#8629=CARTESIAN_POINT('Ctrl Pts',(92.4570000640964,-3.97078332034416,0.0033255119112029));
#8630=CARTESIAN_POINT('Origin',(73.0447820522122,0.,0.));
#8631=CARTESIAN_POINT('',(90.3403333974298,-3.96259069745009,-0.00094416610920911));
#8632=CARTESIAN_POINT('',(90.5072820522123,-3.96576562046892,0.0032106135516634));
#8633=CARTESIAN_POINT('',(73.0447820522122,-3.96875,-4.10839266763092E-13));
#8634=CARTESIAN_POINT('Ctrl Pts',(90.5072820522123,-3.96576562046892,0.00321061355166345));
#8635=CARTESIAN_POINT('Ctrl Pts',(90.5455557570207,-3.95882871231444,-0.900089954804321));
#8636=CARTESIAN_POINT('Ctrl Pts',(90.6396592308354,-3.20563741620691,-3.13149768310236));
#8637=CARTESIAN_POINT('Ctrl Pts',(90.7895924736566,0.492243639519289,-4.6599120176056));
#8638=CARTESIAN_POINT('Ctrl Pts',(90.9570817806758,4.17521467245732,-2.12712653204012));
#8639=CARTESIAN_POINT('Ctrl Pts',(91.1245710876947,4.05905751400097,2.34118289566344));
#8640=CARTESIAN_POINT('Ctrl Pts',(91.2920603947138,0.249466413298239,4.67919297252862));
#8641=CARTESIAN_POINT('Ctrl Pts',(91.4390751606641,-3.29367227435324,2.99416580689908));
#8642=CARTESIAN_POINT('Ctrl Pts',(91.5302601576081,-3.95921382134275,0.832691598517345));
#8643=CARTESIAN_POINT('Ctrl Pts',(91.5656153855456,-3.96419497404471,-0.00256333403586429));
#8644=CARTESIAN_POINT('Ctrl Pts',(90.3403333974298,-3.96259069745009,-0.000944166109208833));
#8645=CARTESIAN_POINT('Ctrl Pts',(90.3657540504659,-3.96387837288311,-0.602107582562329));
#8646=CARTESIAN_POINT('Ctrl Pts',(90.4470044725083,-3.55362928902476,-2.52190045542289));
#8647=CARTESIAN_POINT('Ctrl Pts',(90.584084663557,-0.578055276042246,-4.65004698078105));
#8648=CARTESIAN_POINT('Ctrl Pts',(90.7515739705762,3.58359009673503,-3.01910035578126));
#8649=CARTESIAN_POINT('Ctrl Pts',(90.9190632775952,4.48444073454358,1.35899828774903));
#8650=CARTESIAN_POINT('Ctrl Pts',(91.0865525846143,1.304790942286,4.5005116341675));
#8651=CARTESIAN_POINT('Ctrl Pts',(91.2464204023369,-2.8634060745579,3.59029486786392));
#8652=CARTESIAN_POINT('Ctrl Pts',(91.3504584510532,-3.96335862525385,1.13003881420564));
#8653=CARTESIAN_POINT('Ctrl Pts',(91.3986667307631,-3.97246823586828,-0.00280997941530784));
#8654=CARTESIAN_POINT('Origin',(73.0447820522122,0.,0.));
#8655=CARTESIAN_POINT('',(89.2820000640964,-3.9690716332801,0.00355215784508645));
#8656=CARTESIAN_POINT('',(89.4489487188789,-3.97520890573159,-0.000105091489476044));
#8657=CARTESIAN_POINT('',(73.0447820522122,-3.96875,-4.10839266763092E-13));
#8658=CARTESIAN_POINT('Ctrl Pts',(89.4489487188789,-3.97520890573159,-0.000105091489475756));
#8659=CARTESIAN_POINT('Ctrl Pts',(89.4491918184206,-3.97521113687027,-0.00580729351476086));
#8660=CARTESIAN_POINT('Ctrl Pts',(89.5052646869687,-3.97262415068171,-1.32106406366707));
#8661=CARTESIAN_POINT('Ctrl Pts',(89.617167324523,-2.53692607573313,-3.93968151281212));
#8662=CARTESIAN_POINT('Ctrl Pts',(89.7846566315422,1.9203526326146,-4.27426368987786));
#8663=CARTESIAN_POINT('Ctrl Pts',(89.9521459385612,4.63025632975995,-0.719590617471205));
#8664=CARTESIAN_POINT('Ctrl Pts',(90.1196352455803,3.12697851528032,3.48985525802016));
#8665=CARTESIAN_POINT('Ctrl Pts',(90.2871245525994,-1.22161219883188,4.5237979510226));
#8666=CARTESIAN_POINT('Ctrl Pts',(90.4163401548101,-3.71892401632552,2.14579381908193));
#8667=CARTESIAN_POINT('Ctrl Pts',(90.4897259880143,-3.96894756497898,0.417552597100143));
#8668=CARTESIAN_POINT('Ctrl Pts',(90.5072820522123,-3.96576562046892,0.00321061355166345));
#8669=CARTESIAN_POINT('Ctrl Pts',(89.2820000640964,-3.9690716332801,0.00355215784508672));
#8670=CARTESIAN_POINT('Ctrl Pts',(89.3252198808721,-3.95978931658861,-1.0143213554308));
#8671=CARTESIAN_POINT('Ctrl Pts',(89.4242694666542,-3.04365128022373,-3.36189206530121));
#8672=CARTESIAN_POINT('Ctrl Pts',(89.5791488214426,0.900310895961415,-4.59853511258327));
#8673=CARTESIAN_POINT('Ctrl Pts',(89.7466381284616,4.34616767952069,-1.75154543008276));
#8674=CARTESIAN_POINT('Ctrl Pts',(89.9141274354808,3.83734204230666,2.68921753416258));
#8675=CARTESIAN_POINT('Ctrl Pts',(90.0816167424998,-0.163173340857844,4.68299683371814));
#8676=CARTESIAN_POINT('Ctrl Pts',(90.2236853964828,-3.43057084216195,2.75973770851382));
#8677=CARTESIAN_POINT('Ctrl Pts',(90.3099242814595,-3.9610503329473,0.718189524991144));
#8678=CARTESIAN_POINT('Ctrl Pts',(90.3403333974298,-3.96259069745009,-0.000944166109208833));
#8679=CARTESIAN_POINT('Origin',(73.0447820522122,0.,0.));
#8680=CARTESIAN_POINT('',(88.223666730763,-3.97382271423798,-0.00207988543367732));
#8681=CARTESIAN_POINT('',(88.3906153855456,-3.96547802822572,-0.00312327481737352));
#8682=CARTESIAN_POINT('',(73.0447820522122,-3.96875,-4.10839266763092E-13));
#8683=CARTESIAN_POINT('Ctrl Pts',(88.3906153855456,-3.96547802822572,-0.00312327481737304));
#8684=CARTESIAN_POINT('Ctrl Pts',(88.4086576488269,-3.96864298053677,-0.429018094393009));
#8685=CARTESIAN_POINT('Ctrl Pts',(88.4825296811146,-3.70967706911612,-2.16905097144579));
#8686=CARTESIAN_POINT('Ctrl Pts',(88.6122314824085,-1.18239306112185,-4.53420676431444));
#8687=CARTESIAN_POINT('Ctrl Pts',(88.7797207894278,3.15708129655885,-3.46264667837653));
#8688=CARTESIAN_POINT('Ctrl Pts',(88.9472100964467,4.6238515098096,0.75965883636597));
#8689=CARTESIAN_POINT('Ctrl Pts',(89.1146994034659,1.88326811136568,4.29073251947842));
#8690=CARTESIAN_POINT('Ctrl Pts',(89.2819456109432,-2.56448120676564,3.91810719258513));
#8691=CARTESIAN_POINT('Ctrl Pts',(89.3933620494143,-3.97469873788979,1.30374935835586));
#8692=CARTESIAN_POINT('Ctrl Pts',(89.4489487188789,-3.97520890573159,-0.000105091489475756));
#8693=CARTESIAN_POINT('Ctrl Pts',(88.223666730763,-3.97382271423798,-0.00207988543367638));
#8694=CARTESIAN_POINT('Ctrl Pts',(88.228855942272,-3.97460074042894,-0.123912364854287));
#8695=CARTESIAN_POINT('Ctrl Pts',(88.2898749227873,-3.91438819662648,-1.55573883041568));
#8696=CARTESIAN_POINT('Ctrl Pts',(88.4067236723092,-2.18047806078814,-4.1476017550482));
#8697=CARTESIAN_POINT('Ctrl Pts',(88.574212979328,2.28895303198969,-4.08873805829862));
#8698=CARTESIAN_POINT('Ctrl Pts',(88.7417022863472,4.67561075159403,-0.309433339534459));
#8699=CARTESIAN_POINT('Ctrl Pts',(88.9091915933663,2.80781788150847,3.75143221135632));
#8700=CARTESIAN_POINT('Ctrl Pts',(89.0766809003853,-1.614875957977,4.39877943664814));
#8701=CARTESIAN_POINT('Ctrl Pts',(89.2009503906287,-3.80607569236581,1.90936693291494));
#8702=CARTESIAN_POINT('Ctrl Pts',(89.2693901118658,-3.97177987174111,0.300530195625075));
#8703=CARTESIAN_POINT('Ctrl Pts',(89.2820000640964,-3.9690716332801,0.00355215784508672));
#8704=CARTESIAN_POINT('Origin',(73.0447820522122,0.,0.));
#8705=CARTESIAN_POINT('',(87.1653333974297,-3.96319350967473,-0.00180240263408987));
#8706=CARTESIAN_POINT('',(87.3322820522123,-3.96442879726087,0.0026902431041884));
#8707=CARTESIAN_POINT('',(73.0447820522122,-3.96875,-4.10839266763092E-13));
#8708=CARTESIAN_POINT('Ctrl Pts',(87.3322820522123,-3.96442879726087,0.00269024310418864));
#8709=CARTESIAN_POINT('Ctrl Pts',(87.3681234792332,-3.95910818549169,-0.843925282767195));
#8710=CARTESIAN_POINT('Ctrl Pts',(87.4597946752604,-3.27938659012527,-3.01710310342379));
#8711=CARTESIAN_POINT('Ctrl Pts',(87.6072956402942,0.289976004112983,-4.67685773244287));
#8712=CARTESIAN_POINT('Ctrl Pts',(87.7747849473131,4.07917855433484,-2.3059459348224));
#8713=CARTESIAN_POINT('Ctrl Pts',(87.9422742543323,4.15663850493095,2.16320148663827));
#8714=CARTESIAN_POINT('Ctrl Pts',(88.1097635613514,0.451873185294068,4.66399988817462));
#8715=CARTESIAN_POINT('Ctrl Pts',(88.2592106050891,-3.22068607939857,3.10868133478913));
#8716=CARTESIAN_POINT('Ctrl Pts',(88.3528278798206,-3.95884938902959,0.888865866569467));
#8717=CARTESIAN_POINT('Ctrl Pts',(88.3906153855456,-3.96547802822572,-0.00312327481737304));
#8718=CARTESIAN_POINT('Ctrl Pts',(87.1653333974297,-3.96319350967473,-0.00180240263408953));
#8719=CARTESIAN_POINT('Ctrl Pts',(87.1883217726783,-3.96543626138576,-0.545238984627107));
#8720=CARTESIAN_POINT('Ctrl Pts',(87.2671399169332,-3.6083985865186,-2.40564992743396));
#8721=CARTESIAN_POINT('Ctrl Pts',(87.4017878301947,-0.778891559482246,-4.62065069342133));
#8722=CARTESIAN_POINT('Ctrl Pts',(87.5692771372135,3.44948051298471,-3.17146166342683));
#8723=CARTESIAN_POINT('Ctrl Pts',(87.7367664442328,4.53908736689592,1.16351655241039));
#8724=CARTESIAN_POINT('Ctrl Pts',(87.9042557512518,1.49846953985345,4.43978309494734));
#8725=CARTESIAN_POINT('Ctrl Pts',(88.066555846762,-2.76919203824914,3.69984238148232));
#8726=CARTESIAN_POINT('Ctrl Pts',(88.1730261732656,-3.96623010021758,1.18686079823135));
#8727=CARTESIAN_POINT('Ctrl Pts',(88.223666730763,-3.97382271423798,-0.00207988543367638));
#8728=CARTESIAN_POINT('Origin',(73.0447820522122,0.,0.));
#8729=CARTESIAN_POINT('',(86.1070000640964,-3.96737955141156,0.00351402329782577));
#8730=CARTESIAN_POINT('',(86.2739487188789,-3.97493882611752,0.00093324338624715));
#8731=CARTESIAN_POINT('',(73.0447820522122,-3.96875,-4.10839266763092E-13));
#8732=CARTESIAN_POINT('Ctrl Pts',(86.2739487188789,-3.97493882611752,0.000933243386247009));
#8733=CARTESIAN_POINT('Ctrl Pts',(86.3275893096394,-3.97092371063276,-1.25750325867978));
#8734=CARTESIAN_POINT('Ctrl Pts',(86.4370596694064,-2.6471458759135,-3.83301135212251));
#8735=CARTESIAN_POINT('Ctrl Pts',(86.6023597981797,1.7334463653411,-4.35341797108391));
#8736=CARTESIAN_POINT('Ctrl Pts',(86.7698491051987,4.59474916176048,-0.919437041331279));
#8737=CARTESIAN_POINT('Ctrl Pts',(86.9373384122179,3.27517927238433,3.35116174873949));
#8738=CARTESIAN_POINT('Ctrl Pts',(87.1048277192368,-1.02455494782308,4.5724579266913));
#8739=CARTESIAN_POINT('Ctrl Pts',(87.2364755992351,-3.67140987877257,2.26215094425435));
#8740=CARTESIAN_POINT('Ctrl Pts',(87.3122937102269,-3.96739603981938,0.47483775696838));
#8741=CARTESIAN_POINT('Ctrl Pts',(87.3322820522123,-3.96442879726087,0.00269024310418864));
#8742=CARTESIAN_POINT('Ctrl Pts',(86.1070000640964,-3.96737955141156,0.0035140232978258));
#8743=CARTESIAN_POINT('Ctrl Pts',(86.1477876030846,-3.9590346583871,-0.9581231290712));
#8744=CARTESIAN_POINT('Ctrl Pts',(86.2444049110792,-3.1253503766273,-3.24901199396521));
#8745=CARTESIAN_POINT('Ctrl Pts',(86.3968519880801,0.700318456568796,-4.63321043677455));
#8746=CARTESIAN_POINT('Ctrl Pts',(86.5643412950992,4.26623638905772,-1.93812073017321));
#8747=CARTESIAN_POINT('Ctrl Pts',(86.7318306021183,3.9502033026309,2.52051160678369));
#8748=CARTESIAN_POINT('Ctrl Pts',(86.8993199091373,0.0397852977070385,4.68566985842301));
#8749=CARTESIAN_POINT('Ctrl Pts',(87.0438208409079,-3.36514974078574,2.87524198487157));
#8750=CARTESIAN_POINT('Ctrl Pts',(87.132492003672,-3.95998949498269,0.774555847073451));
#8751=CARTESIAN_POINT('Ctrl Pts',(87.1653333974297,-3.96319350967473,-0.00180240263408953));
#8752=CARTESIAN_POINT('Origin',(73.0447820522122,0.,0.));
#8753=CARTESIAN_POINT('',(85.0486667307631,-3.97478647022473,-0.00116584238653683));
#8754=CARTESIAN_POINT('',(85.2156153855456,-3.96699920481957,-0.00346812739152993));
#8755=CARTESIAN_POINT('',(73.0447820522122,-3.96875,-4.10839266763092E-13));
#8756=CARTESIAN_POINT('Ctrl Pts',(85.2156153855455,-3.96699920481957,-0.00346812739152977));
#8757=CARTESIAN_POINT('Ctrl Pts',(85.2312253710394,-3.9701271390701,-0.371590363698427));
#8758=CARTESIAN_POINT('Ctrl Pts',(85.3026651255396,-3.75470286066849,-2.0527260743823));
#8759=CARTESIAN_POINT('Ctrl Pts',(85.4299346490461,-1.37764569709891,-4.47874722056687));
#8760=CARTESIAN_POINT('Ctrl Pts',(85.5974239560652,3.0041632824441,-3.59612114713693));
#8761=CARTESIAN_POINT('Ctrl Pts',(85.7649132630843,4.65241189360609,0.558701982011273));
#8762=CARTESIAN_POINT('Ctrl Pts',(85.9324025701033,2.06731911348409,4.20514875069765));
#8763=CARTESIAN_POINT('Ctrl Pts',(86.0998918771224,-2.39887701093383,4.02522961070344));
#8764=CARTESIAN_POINT('Ctrl Pts',(86.213740593381,-3.95098917456334,1.4132901908714));
#8765=CARTESIAN_POINT('Ctrl Pts',(86.2717595406331,-3.97510269089508,0.0522925176778244));
#8766=CARTESIAN_POINT('Ctrl Pts',(86.2739487188789,-3.97493882611752,0.000933243386247009));
#8767=CARTESIAN_POINT('Ctrl Pts',(85.0486667307631,-3.97478647022473,-0.00116584238653631));
#8768=CARTESIAN_POINT('Ctrl Pts',(85.0514236644845,-3.97503858705613,-0.0658515906554392));
#8769=CARTESIAN_POINT('Ctrl Pts',(85.1100103672124,-3.94436777223071,-1.44022332085691));
#8770=CARTESIAN_POINT('Ctrl Pts',(85.2244268389466,-2.35805169304712,-4.04928106025811));
#8771=CARTESIAN_POINT('Ctrl Pts',(85.3919161459656,2.10973547078508,-4.18402929427589));
#8772=CARTESIAN_POINT('Ctrl Pts',(85.5594054529847,4.65782362744017,-0.511628720565475));
#8773=CARTESIAN_POINT('Ctrl Pts',(85.7268947600037,2.96764612613796,3.62631512172698));
#8774=CARTESIAN_POINT('Ctrl Pts',(85.894384067023,-1.42286390542218,4.46458768518373));
#8775=CARTESIAN_POINT('Ctrl Pts',(86.0210858350537,-3.76477370815308,2.02558326012544));
#8776=CARTESIAN_POINT('Ctrl Pts',(86.0919578340782,-3.97045710410203,0.358160751165195));
#8777=CARTESIAN_POINT('Ctrl Pts',(86.1070000640964,-3.96737955141156,0.0035140232978258));
#8778=CARTESIAN_POINT('Origin',(73.0447820522122,0.,0.));
#8779=CARTESIAN_POINT('',(83.9903333974298,-3.9641570283979,-0.00254082259245281));
#8780=CARTESIAN_POINT('',(84.1572820522123,-3.96338763911034,0.00198750657534593));
#8781=CARTESIAN_POINT('',(73.0447820522122,-3.96875,-4.10839266763092E-13));
#8782=CARTESIAN_POINT('Ctrl Pts',(84.1572820522123,-3.96338763911034,0.00198750657534594));
#8783=CARTESIAN_POINT('Ctrl Pts',(84.1906912014457,-3.95978296584885,-0.787695341446297));
#8784=CARTESIAN_POINT('Ctrl Pts',(84.2799301196855,-3.34935300432391,-2.90214532004246));
#8785=CARTESIAN_POINT('Ctrl Pts',(84.4249988069316,0.0871642670565068,-4.68502793193585));
#8786=CARTESIAN_POINT('Ctrl Pts',(84.5924881139508,3.97548844210186,-2.48043866668484));
#8787=CARTESIAN_POINT('Ctrl Pts',(84.7599774209698,4.24642014257932,1.9811613526332));
#8788=CARTESIAN_POINT('Ctrl Pts',(84.9274667279889,0.653432103046516,4.64005504484363));
#8789=CARTESIAN_POINT('Ctrl Pts',(85.0793460495141,-3.14384921632806,3.22254157615712));
#8790=CARTESIAN_POINT('Ctrl Pts',(85.175395602033,-3.95893995079608,0.945014281914011));
#8791=CARTESIAN_POINT('Ctrl Pts',(85.2156153855455,-3.96699920481957,-0.00346812739152977));
#8792=CARTESIAN_POINT('Ctrl Pts',(83.9903333974298,-3.9641570283979,-0.00254082259245246));
#8793=CARTESIAN_POINT('Ctrl Pts',(84.0108894948909,-3.96702649059957,-0.488183074464591));
#8794=CARTESIAN_POINT('Ctrl Pts',(84.0872753613584,-3.65986279650672,-2.28931254822536));
#8795=CARTESIAN_POINT('Ctrl Pts',(84.219490996832,-0.97826636104911,-4.58258440390215));
#8796=CARTESIAN_POINT('Ctrl Pts',(84.3869803038513,3.30889846384542,-3.31787218681023));
#8797=CARTESIAN_POINT('Ctrl Pts',(84.5544696108702,4.58521705524031,0.965851669968393));
#8798=CARTESIAN_POINT('Ctrl Pts',(84.7219589178894,1.68933645364314,4.37072388037037));
#8799=CARTESIAN_POINT('Ctrl Pts',(84.886691291187,-2.67074242799831,3.80798725931741));
#8800=CARTESIAN_POINT('Ctrl Pts',(84.9955938954782,-3.96993305102157,1.24407847974412));
#8801=CARTESIAN_POINT('Ctrl Pts',(85.0486667307631,-3.97478647022473,-0.00116584238653631));
#8802=CARTESIAN_POINT('Origin',(73.0447820522122,0.,0.));
#8803=CARTESIAN_POINT('',(82.9320000640964,-3.96581480482491,0.00322439829302731));
#8804=CARTESIAN_POINT('',(83.0989487188788,-3.97408812184296,0.0018807273087504));
#8805=CARTESIAN_POINT('',(73.0447820522122,-3.96875,-4.10839266763092E-13));
#8806=CARTESIAN_POINT('Ctrl Pts',(83.0989487188788,-3.97408812184296,0.00188072730875047));
#8807=CARTESIAN_POINT('Ctrl Pts',(83.1501570318519,-3.9670176952052,-1.20017749285163));
#8808=CARTESIAN_POINT('Ctrl Pts',(83.2571951138316,-2.74659247719471,-3.72521760004062));
#8809=CARTESIAN_POINT('Ctrl Pts',(83.4200629648169,1.54328753190602,-4.42440368030926));
#8810=CARTESIAN_POINT('Ctrl Pts',(83.5875522718364,4.5506205990891,-1.11755827392429));
#8811=CARTESIAN_POINT('Ctrl Pts',(83.7550415788553,3.41723462017294,3.20618026367237));
#8812=CARTESIAN_POINT('Ctrl Pts',(83.9225308858744,-0.825575264478656,4.61253832668647));
#8813=CARTESIAN_POINT('Ctrl Pts',(84.05661104366,-3.62070390902415,2.37849907820253));
#8814=CARTESIAN_POINT('Ctrl Pts',(84.1348614324393,-3.96580670725351,0.531937513771429));
#8815=CARTESIAN_POINT('Ctrl Pts',(84.1572820522123,-3.96338763911034,0.00198750657534594));
#8816=CARTESIAN_POINT('Ctrl Pts',(82.9320000640964,-3.96581480482491,0.00322439829302756));
#8817=CARTESIAN_POINT('Ctrl Pts',(82.9703553252971,-3.95882711771097,-0.901972645909376));
#8818=CARTESIAN_POINT('Ctrl Pts',(83.0645403555041,-3.2030980355045,-3.13532234621704));
#8819=CARTESIAN_POINT('Ctrl Pts',(83.2145551547178,0.499011969014512,-4.65919219895763));
#8820=CARTESIAN_POINT('Ctrl Pts',(83.3820444617366,4.17830011134652,-2.12105942197974));
#8821=CARTESIAN_POINT('Ctrl Pts',(83.5495337687558,4.05565256718464,2.34707629751062));
#8822=CARTESIAN_POINT('Ctrl Pts',(83.7170230757749,0.242669284494185,4.67955088768255));
#8823=CARTESIAN_POINT('Ctrl Pts',(83.8639562853328,-3.29605384042193,2.99031534253484));
#8824=CARTESIAN_POINT('Ctrl Pts',(83.9550597258845,-3.959233113856,0.830807302627488));
#8825=CARTESIAN_POINT('Ctrl Pts',(83.9903333974298,-3.9641570283979,-0.00254082259245246));
#8826=CARTESIAN_POINT('Origin',(73.0447820522122,0.,0.));
#8827=CARTESIAN_POINT('',(81.873666730763,-3.97520616141411,-0.000140328321075467));
#8828=CARTESIAN_POINT('',(82.0406153855455,-3.96867065624537,-0.00356668729390831));
#8829=CARTESIAN_POINT('',(73.0447820522122,-3.96875,-4.10839266763092E-13));
#8830=CARTESIAN_POINT('Ctrl Pts',(82.0406153855455,-3.96867065624537,-0.00356668729390795));
#8831=CARTESIAN_POINT('Ctrl Pts',(82.0537930932519,-3.97148539159384,-0.313996266888609));
#8832=CARTESIAN_POINT('Ctrl Pts',(82.1228005699646,-3.79669925955763,-1.93648425285867));
#8833=CARTESIAN_POINT('Ctrl Pts',(82.2476378156836,-1.57031337642494,-4.4148839432415));
#8834=CARTESIAN_POINT('Ctrl Pts',(82.4151271227027,2.84560838224604,-3.72284800486962));
#8835=CARTESIAN_POINT('Ctrl Pts',(82.5826164297219,4.67224268670378,0.3566968026402));
#8836=CARTESIAN_POINT('Ctrl Pts',(82.7501057367407,2.24749108465355,4.11167461709625));
#8837=CARTESIAN_POINT('Ctrl Pts',(82.9175950437602,-2.22230666825049,4.1253408834568));
#8838=CARTESIAN_POINT('Ctrl Pts',(83.0338760378059,-3.92162237958999,1.52875551670549));
#8839=CARTESIAN_POINT('Ctrl Pts',(83.0943272628455,-3.97472621483892,0.110364270143812));
#8840=CARTESIAN_POINT('Ctrl Pts',(83.0989487188788,-3.97408812184296,0.00188072730875047));
#8841=CARTESIAN_POINT('Ctrl Pts',(81.8736667307631,-3.97520616141411,-0.000140328321074999));
#8842=CARTESIAN_POINT('Ctrl Pts',(81.873991386697,-3.97521012478093,-0.00775555150819479));
#8843=CARTESIAN_POINT('Ctrl Pts',(81.9301458116374,-3.97175020506519,-1.32492622653714));
#8844=CARTESIAN_POINT('Ctrl Pts',(82.0421300055841,-2.53120077593259,-3.94336246418788));
#8845=CARTESIAN_POINT('Ctrl Pts',(82.2096193126032,1.92655929036014,-4.27146979303078));
#8846=CARTESIAN_POINT('Ctrl Pts',(82.3771086196222,4.63129675823398,-0.712864102910859));
#8847=CARTESIAN_POINT('Ctrl Pts',(82.5445979266413,3.12190600394933,3.49439376638532));
#8848=CARTESIAN_POINT('Ctrl Pts',(82.7120872336604,-1.22818205067104,4.52201876847685));
#8849=CARTESIAN_POINT('Ctrl Pts',(82.8412212794788,-3.72046301701938,2.14189278432346));
#8850=CARTESIAN_POINT('Ctrl Pts',(82.9145255562908,-3.96899836789274,0.415628650522889));
#8851=CARTESIAN_POINT('Ctrl Pts',(82.9320000640964,-3.96581480482491,0.00322439829302756));
#8852=CARTESIAN_POINT('Origin',(73.0447820522122,0.,0.));
#8853=CARTESIAN_POINT('',(80.8153333974297,-3.96543075761921,-0.00310776878558905));
#8854=CARTESIAN_POINT('',(80.9822820522122,-3.96269713818528,0.00115225484714665));
#8855=CARTESIAN_POINT('',(73.0447820522122,-3.96875,-4.10839266763092E-13));
#8856=CARTESIAN_POINT('Ctrl Pts',(80.9822820522122,-3.96269713818528,0.00115225484714682));
#8857=CARTESIAN_POINT('Ctrl Pts',(81.0132589236582,-3.96077923108138,-0.731358860291098));
#8858=CARTESIAN_POINT('Ctrl Pts',(81.1000655641105,-3.41562392927438,-2.78673257207323));
#8859=CARTESIAN_POINT('Ctrl Pts',(81.2427019735693,-0.115811021377698,-4.68440734136128));
#8860=CARTESIAN_POINT('Ctrl Pts',(81.4101912805881,3.86433888996382,-2.65027720738482));
#8861=CARTESIAN_POINT('Ctrl Pts',(81.5776805876074,4.32823397543431,1.79540385049343));
#8862=CARTESIAN_POINT('Ctrl Pts',(81.7451698946263,0.853764948185291,4.60740379668648));
#8863=CARTESIAN_POINT('Ctrl Pts',(81.8994814939392,-3.06307956634302,3.3356222962608));
#8864=CARTESIAN_POINT('Ctrl Pts',(81.9979633242455,-3.95956025045237,1.00119542712499));
#8865=CARTESIAN_POINT('Ctrl Pts',(82.0406153855455,-3.96867065624537,-0.00356668729390795));
#8866=CARTESIAN_POINT('Ctrl Pts',(80.8153333974297,-3.9654307576192,-0.00310776878558985));
#8867=CARTESIAN_POINT('Ctrl Pts',(80.8334572171033,-3.96859161685811,-0.430940653862831));
#8868=CARTESIAN_POINT('Ctrl Pts',(80.9074108057833,-3.70811382132026,-2.17295237118825));
#8869=CARTESIAN_POINT('Ctrl Pts',(81.0371941634697,-1.17580558461439,-4.53591954505886));
#8870=CARTESIAN_POINT('Ctrl Pts',(81.2046834704886,3.16210773630061,-3.45805719386958));
#8871=CARTESIAN_POINT('Ctrl Pts',(81.3721727775078,4.62274323446282,0.766374503930213));
#8872=CARTESIAN_POINT('Ctrl Pts',(81.5396620845268,1.87703356730924,4.29346362267612));
#8873=CARTESIAN_POINT('Ctrl Pts',(81.706826735612,-2.56800120527708,3.91456288380908));
#8874=CARTESIAN_POINT('Ctrl Pts',(81.8181616176907,-3.97452856060593,1.30180360625973));
#8875=CARTESIAN_POINT('Ctrl Pts',(81.8736667307631,-3.97520616141411,-0.000140328321074999));
#8876=CARTESIAN_POINT('Origin',(73.0447820522122,0.,0.));
#8877=CARTESIAN_POINT('',(79.7570000640964,-3.96446924306102,0.00271090097985122));
#8878=CARTESIAN_POINT('',(79.9239487188789,-3.97281147716045,0.00265889188302577));
#8879=CARTESIAN_POINT('',(73.0447820522122,-3.96875,-4.10839266763092E-13));
#8880=CARTESIAN_POINT('Ctrl Pts',(79.9239487188789,-3.97281147716045,0.00265889188302577));
#8881=CARTESIAN_POINT('Ctrl Pts',(79.9727247540645,-3.96395783417343,-1.14327265515754));
#8882=CARTESIAN_POINT('Ctrl Pts',(80.0773305582564,-2.8417898791282,-3.61598293165399));
#8883=CARTESIAN_POINT('Ctrl Pts',(80.2377661314547,1.35023293842321,-4.48708762389827));
#8884=CARTESIAN_POINT('Ctrl Pts',(80.4052554384738,4.49795344263644,-1.3135825670034));
#8885=CARTESIAN_POINT('Ctrl Pts',(80.5727447454928,3.55287801213224,3.05518283632336));
#8886=CARTESIAN_POINT('Ctrl Pts',(80.7402340525119,-0.625046506306802,4.64396395307223));
#8887=CARTESIAN_POINT('Ctrl Pts',(80.8767464880851,-3.56671435023439,2.49477603427471));
#8888=CARTESIAN_POINT('Ctrl Pts',(80.9574291546518,-3.96423588456471,0.588849554690602));
#8889=CARTESIAN_POINT('Ctrl Pts',(80.9822820522122,-3.96269713818528,0.00115225484714682));
#8890=CARTESIAN_POINT('Ctrl Pts',(79.7570000640964,-3.96446924306102,0.00271090097985101));
#8891=CARTESIAN_POINT('Ctrl Pts',(79.7929230475096,-3.95909204437552,-0.845809344955338));
#8892=CARTESIAN_POINT('Ctrl Pts',(79.8846757999293,-3.27697553121347,-3.02094864559479));
#8893=CARTESIAN_POINT('Ctrl Pts',(80.032258321355,0.296769156290057,-4.67643164821721));
#8894=CARTESIAN_POINT('Ctrl Pts',(80.1997476283743,4.08252384642615,-2.30001824674852));
#8895=CARTESIAN_POINT('Ctrl Pts',(80.3672369353933,4.15349197522231,2.16923703262104));
#8896=CARTESIAN_POINT('Ctrl Pts',(80.5347262424123,0.445097936809096,4.66465140377808));
#8897=CARTESIAN_POINT('Ctrl Pts',(80.6840917297579,-3.22319533629547,3.10485150926155));
#8898=CARTESIAN_POINT('Ctrl Pts',(80.777627448097,-3.9588547046427,0.88698302764329));
#8899=CARTESIAN_POINT('Ctrl Pts',(80.8153333974297,-3.9654307576192,-0.00310776878558985));
#8900=CARTESIAN_POINT('Origin',(73.0447820522122,0.,0.));
#8901=CARTESIAN_POINT('',(78.6986667307631,-3.97495822072444,0.000899384355832079));
#8902=CARTESIAN_POINT('',(78.8656153855456,-3.97038802851853,-0.00340262987801933));
#8903=CARTESIAN_POINT('',(73.0447820522122,-3.96875,-4.10839266763092E-13));
#8904=CARTESIAN_POINT('Ctrl Pts',(78.8656153855456,-3.97038802851853,-0.00340262987801949));
#8905=CARTESIAN_POINT('Ctrl Pts',(78.8763608154644,-3.97267697458941,-0.256253454012208));
#8906=CARTESIAN_POINT('Ctrl Pts',(78.9429360143896,-3.8357540982908,-1.82036601749888));
#8907=CARTESIAN_POINT('Ctrl Pts',(79.065340982321,-1.76003458552832,-4.34273676176006));
#8908=CARTESIAN_POINT('Ctrl Pts',(79.2328302893404,2.68171410172883,-3.84258946710639));
#8909=CARTESIAN_POINT('Ctrl Pts',(79.4003195963591,4.6833066794353,0.154022332581167));
#8910=CARTESIAN_POINT('Ctrl Pts',(79.5678089033785,2.42344595773958,4.01048550943476));
#8911=CARTESIAN_POINT('Ctrl Pts',(79.7352982103974,-2.04156648246805,4.21771153952704));
#8912=CARTESIAN_POINT('Ctrl Pts',(79.8540114822309,-3.88960149513591,1.64443102927543));
#8913=CARTESIAN_POINT('Ctrl Pts',(79.9168949850581,-3.97409184447069,0.168377488708408));
#8914=CARTESIAN_POINT('Ctrl Pts',(79.9239487188789,-3.97281147716045,0.00265889188302577));
#8915=CARTESIAN_POINT('Ctrl Pts',(78.6986667307631,-3.97495822072444,0.000899384355832027));
#8916=CARTESIAN_POINT('Ctrl Pts',(78.7523888779159,-3.97107011656311,-1.25943406802524));
#8917=CARTESIAN_POINT('Ctrl Pts',(78.8619407940752,-2.64373708770944,-3.83659888994191));
#8918=CARTESIAN_POINT('Ctrl Pts',(79.0273224792406,1.73976819338591,-4.35089548826393));
#8919=CARTESIAN_POINT('Ctrl Pts',(79.1948117862598,4.5960799186112,-0.912761895211113));
#8920=CARTESIAN_POINT('Ctrl Pts',(79.3623010932788,3.2703080678004,3.35591567615466));
#8921=CARTESIAN_POINT('Ctrl Pts',(79.529790400298,-1.03119568640402,4.57096492570699));
#8922=CARTESIAN_POINT('Ctrl Pts',(79.6613567239037,-3.67305432406073,2.25824923837563));
#8923=CARTESIAN_POINT('Ctrl Pts',(79.7370932785032,-3.96744902734265,0.472919914885131));
#8924=CARTESIAN_POINT('Ctrl Pts',(79.7570000640964,-3.96446924306102,0.00271090097985101));
#8925=CARTESIAN_POINT('Origin',(73.0447820522122,0.,0.));
#8926=CARTESIAN_POINT('',(77.6403333974297,-3.96694525050465,-0.00346035837147873));
#8927=CARTESIAN_POINT('',(77.8072820522122,-3.96239275275613,0.000241017124700969));
#8928=CARTESIAN_POINT('',(73.0447820522122,-3.96875,-4.10839266763092E-13));
#8929=CARTESIAN_POINT('Ctrl Pts',(77.8072820522122,-3.96239275275613,0.000241017124700885));
#8930=CARTESIAN_POINT('Ctrl Pts',(77.8358266458707,-3.96202476903025,-0.674883524491887));
#8931=CARTESIAN_POINT('Ctrl Pts',(77.9202010085355,-3.4782887115833,-2.67096469036072));
#8932=CARTESIAN_POINT('Ctrl Pts',(78.0604051402067,-0.318569006102588,-4.67499706960582));
#8933=CARTESIAN_POINT('Ctrl Pts',(78.2278944472258,3.74593845389551,-2.81514290719053));
#8934=CARTESIAN_POINT('Ctrl Pts',(78.3953837542449,4.40192649164485,1.60627754211177));
#8935=CARTESIAN_POINT('Ctrl Pts',(78.5628730612639,1.05249582445596,4.56610740188116));
#8936=CARTESIAN_POINT('Ctrl Pts',(78.7196169383641,-2.97829873546034,3.44779152646148));
#8937=CARTESIAN_POINT('Ctrl Pts',(78.820531046458,-3.96078435313356,1.05747742610126));
#8938=CARTESIAN_POINT('Ctrl Pts',(78.8656153855456,-3.97038802851853,-0.00340262987801949));
#8939=CARTESIAN_POINT('Ctrl Pts',(77.6403333974297,-3.96694525050465,-0.00346035837147901));
#8940=CARTESIAN_POINT('Ctrl Pts',(77.6560249393158,-3.97007923854559,-0.373518795794246));
#8941=CARTESIAN_POINT('Ctrl Pts',(77.7275462502083,-3.75324294587763,-2.05662596994668));
#8942=CARTESIAN_POINT('Ctrl Pts',(77.8548973301072,-1.3711384097138,-4.48074328527017));
#8943=CARTESIAN_POINT('Ctrl Pts',(78.0223866371261,3.00938367803536,-3.59175384599341));
#8944=CARTESIAN_POINT('Ctrl Pts',(78.1898759441454,4.65159553477052,0.565459445670238));
#8945=CARTESIAN_POINT('Ctrl Pts',(78.3573652511643,2.06120867216333,4.20814723864878));
#8946=CARTESIAN_POINT('Ctrl Pts',(78.5248545581835,-2.40472141992828,4.02174090914329));
#8947=CARTESIAN_POINT('Ctrl Pts',(78.6386217180497,-3.95192880893686,1.4094223321187));
#8948=CARTESIAN_POINT('Ctrl Pts',(78.6965591089095,-3.97511075843437,0.050344659121072));
#8949=CARTESIAN_POINT('Ctrl Pts',(78.6986667307631,-3.97495822072444,0.000899384355832027));
#8950=CARTESIAN_POINT('Origin',(73.0447820522122,0.,0.));
#8951=CARTESIAN_POINT('',(76.5820000640964,-3.96340732379332,0.00203673152180062));
#8952=CARTESIAN_POINT('',(76.7489487188789,-3.97125648760866,0.00321799934434852));
#8953=CARTESIAN_POINT('',(73.0447820522122,-3.96875,-4.10839266763092E-13));
#8954=CARTESIAN_POINT('Ctrl Pts',(76.7489487188789,-3.97125648760866,0.00321799934434826));
#8955=CARTESIAN_POINT('Ctrl Pts',(76.7952924762769,-3.96167939898907,-1.08668061945271));
#8956=CARTESIAN_POINT('Ctrl Pts',(76.8974660026814,-2.93279899559863,-3.50547381449112));
#8957=CARTESIAN_POINT('Ctrl Pts',(77.0554692980923,1.15464486915952,-4.54134892492803));
#8958=CARTESIAN_POINT('Ctrl Pts',(77.2229586051112,4.43684649216151,-1.50714376233198));
#8959=CARTESIAN_POINT('Ctrl Pts',(77.3904479121304,3.68185494419516,2.8984536307935));
#8960=CARTESIAN_POINT('Ctrl Pts',(77.5579372191495,-0.423344942904035,4.66667541455828));
#8961=CARTESIAN_POINT('Ctrl Pts',(77.6968819325101,-3.50934901946654,2.61091163483654));
#8962=CARTESIAN_POINT('Ctrl Pts',(77.7799968768643,-3.96274450064246,0.645578334589518));
#8963=CARTESIAN_POINT('Ctrl Pts',(77.8072820522122,-3.96239275275613,0.000241017124700885));
#8964=CARTESIAN_POINT('Ctrl Pts',(76.5820000640964,-3.96340732379332,0.00203673152180048));
#8965=CARTESIAN_POINT('Ctrl Pts',(76.6154907697221,-3.95974885929359,-0.789568373245937));
#8966=CARTESIAN_POINT('Ctrl Pts',(76.7048112443542,-3.34708273705454,-2.90604413054571));
#8967=CARTESIAN_POINT('Ctrl Pts',(76.8499614879926,0.0939792462890116,-4.68487346091533));
#8968=CARTESIAN_POINT('Ctrl Pts',(77.0174507950118,3.9790823597631,-2.47467306941385));
#8969=CARTESIAN_POINT('Ctrl Pts',(77.1849401020308,4.24354045361218,1.98733341519075));
#8970=CARTESIAN_POINT('Ctrl Pts',(77.3524294090499,0.646690153391397,4.64099636386739));
#8971=CARTESIAN_POINT('Ctrl Pts',(77.5042271741829,-3.1464884727734,3.21873680013792));
#8972=CARTESIAN_POINT('Ctrl Pts',(77.6001951703095,-3.95892865629787,0.943131743083547));
#8973=CARTESIAN_POINT('Ctrl Pts',(77.6403333974297,-3.96694525050465,-0.00346035837147901));
#8974=CARTESIAN_POINT('Origin',(73.0447820522122,0.,0.));
#8975=CARTESIAN_POINT('',(75.5236667307631,-3.97344267433394,0.00300565485589988));
#8976=CARTESIAN_POINT('',(75.6906153855455,-3.97203085734017,-0.00290119714995032));
#8977=CARTESIAN_POINT('',(73.0447820522122,-3.96875,-4.10839266763092E-13));
#8978=CARTESIAN_POINT('',(75.342557724821,-1.8872933839096,3.49128919534762));
#8979=CARTESIAN_POINT('Ctrl Pts',(75.342557724821,-1.8872933839096,3.49128919534762));
#8980=CARTESIAN_POINT('Ctrl Pts',(75.3983874938273,-3.04449504617051,2.86573831175296));
#8981=CARTESIAN_POINT('Ctrl Pts',(75.4587571624747,-3.92241670625081,1.52403516311381));
#8982=CARTESIAN_POINT('Ctrl Pts',(75.5191268311221,-3.97408386750059,0.109459130694996));
#8983=CARTESIAN_POINT('Ctrl Pts',(75.5236667307631,-3.97344267433394,0.0030056548558996));
#8984=CARTESIAN_POINT('',(75.3425577248209,1.88433026752062,3.49313140215104));
#8985=CARTESIAN_POINT('Origin',(75.342557724821,0.,0.));
#8986=CARTESIAN_POINT('Ctrl Pts',(75.3425577248209,1.88433026752062,3.49313140215104));
#8987=CARTESIAN_POINT('Ctrl Pts',(75.3552305591811,1.62306428446166,3.63777505635095));
#8988=CARTESIAN_POINT('Ctrl Pts',(75.4237331625476,0.127158115454225,4.25847409842879));
#8989=CARTESIAN_POINT('Ctrl Pts',(75.5397523827892,-2.8894493037692,3.55765941766253));
#8990=CARTESIAN_POINT('Ctrl Pts',(75.6430987686705,-3.9626869925898,1.11374971637242));
#8991=CARTESIAN_POINT('Ctrl Pts',(75.6906153855455,-3.97203085734017,-0.00290119714995075));
#8992=CARTESIAN_POINT('Origin',(93.8044,5.12956166756098E-16,0.));
#8993=CARTESIAN_POINT('',(93.8044,-3.4544,-4.23041990297461E-16));
#8994=CARTESIAN_POINT('Origin',(93.8044,0.,0.));
#8995=CARTESIAN_POINT('Origin',(93.8044,0.,0.));
#8996=CARTESIAN_POINT('Ctrl Pts',(93.8044,3.25944077490413,1.14408268708708));
#8997=CARTESIAN_POINT('Ctrl Pts',(93.8044,3.30370182902396,1.04545417171708));
#8998=CARTESIAN_POINT('Ctrl Pts',(93.8044,3.34284347050657,0.944859526825618));
#8999=CARTESIAN_POINT('Ctrl Pts',(93.8044,3.37701350822368,0.842684008101753));
#9000=CARTESIAN_POINT('Ctrl Pts',(93.8044,3.41201453172657,0.738023669067848));
#9001=CARTESIAN_POINT('Ctrl Pts',(93.8044,3.44179939777699,0.631704043659911));
#9002=CARTESIAN_POINT('Ctrl Pts',(93.8044,3.46648177007704,0.524108164188268));
#9003=CARTESIAN_POINT('Ctrl Pts',(93.8044,3.49162219305062,0.414515541273143));
#9004=CARTESIAN_POINT('Ctrl Pts',(93.8044,3.51146916062601,0.303598127467765));
#9005=CARTESIAN_POINT('Ctrl Pts',(93.8044,3.52609364298277,0.191739006411684));
#9006=CARTESIAN_POINT('Ctrl Pts',(93.8044,3.5286056838143,0.17252501492684));
#9007=CARTESIAN_POINT('Ctrl Pts',(93.8044,3.53096351737855,0.153283203416008));
#9008=CARTESIAN_POINT('Ctrl Pts',(93.8044,3.53316735501456,0.134015475734087));
#9009=CARTESIAN_POINT('Ctrl Pts',(93.8044,3.53530980696597,0.11528443126119));
#9010=CARTESIAN_POINT('Ctrl Pts',(93.8044,3.5373057763528,0.0965369355126364));
#9011=CARTESIAN_POINT('Ctrl Pts',(93.8044,3.539155377505,0.0777797908629161));
#9012=CARTESIAN_POINT('Ctrl Pts',(93.8044,3.55040037324356,-0.0362577741564758));
#9013=CARTESIAN_POINT('Ctrl Pts',(93.8044,3.5562458585282,-0.150707951384351));
#9014=CARTESIAN_POINT('Ctrl Pts',(93.8044,3.55681577918696,-0.265159368763883));
#9015=CARTESIAN_POINT('Ctrl Pts',(93.8044,3.55739270972121,-0.381018508731895));
#9016=CARTESIAN_POINT('Ctrl Pts',(93.8044,3.55256361134374,-0.496879755034307));
#9017=CARTESIAN_POINT('Ctrl Pts',(93.8044,3.54240581757772,-0.612333394534078));
#9018=CARTESIAN_POINT('Ctrl Pts',(93.8044,3.53584543270908,-0.68689882941604));
#9019=CARTESIAN_POINT('Ctrl Pts',(93.8044,3.52706130454575,-0.761294558717738));
#9020=CARTESIAN_POINT('Ctrl Pts',(93.8044,3.51606280513667,-0.835411364968679));
#9021=CARTESIAN_POINT('Ctrl Pts',(93.8044,3.51139999040036,-0.866833191123442));
#9022=CARTESIAN_POINT('Ctrl Pts',(93.8044,3.50633906785472,-0.898204884631247));
#9023=CARTESIAN_POINT('Ctrl Pts',(93.8044,3.50088026190799,-0.929518090387137));
#9024=CARTESIAN_POINT('Ctrl Pts',(93.8044,3.49775496561313,-0.947445645769051));
#9025=CARTESIAN_POINT('Ctrl Pts',(93.8044,3.4944990202265,-0.965354850221281));
#9026=CARTESIAN_POINT('Ctrl Pts',(93.8044,3.49111569524411,-0.983227940624935));
#9027=CARTESIAN_POINT('Ctrl Pts',(93.8044,3.4690454343486,-1.09981850472082));
#9028=CARTESIAN_POINT('Ctrl Pts',(93.8044,3.44153185396965,-1.21503326772926));
#9029=CARTESIAN_POINT('Ctrl Pts',(93.8044,3.40868809088207,-1.32844742744932));
#9030=CARTESIAN_POINT('Ctrl Pts',(93.8044,3.37588600130194,-1.44171768265341));
#9031=CARTESIAN_POINT('Ctrl Pts',(93.8044,3.33776721958986,-1.55319282835126));
#9032=CARTESIAN_POINT('Ctrl Pts',(93.8044,3.29439245272803,-1.66245456336488));
#9033=CARTESIAN_POINT('Ctrl Pts',(93.8044,3.25093502747342,-1.77192451619872));
#9034=CARTESIAN_POINT('Ctrl Pts',(93.8044,3.20220157692753,-1.87917356251577));
#9035=CARTESIAN_POINT('Ctrl Pts',(93.8044,3.14820100366361,-1.98377184954477));
#9036=CARTESIAN_POINT('Ctrl Pts',(93.8044,3.12120071703165,-2.03607099305928));
#9037=CARTESIAN_POINT('Ctrl Pts',(93.8044,3.09288283468518,-2.08770721520033));
#9038=CARTESIAN_POINT('Ctrl Pts',(93.8044,3.06324357590169,-2.13862478061915));
#9039=CARTESIAN_POINT('Ctrl Pts',(93.8044,3.04731869343744,-2.16598228812578));
#9040=CARTESIAN_POINT('Ctrl Pts',(93.8044,3.03101229920686,-2.19313230536482));
#9041=CARTESIAN_POINT('Ctrl Pts',(93.8044,3.01432341729309,-2.22006596460196));
#9042=CARTESIAN_POINT('Ctrl Pts',(93.8044,3.00471242017603,-2.23557684919071));
#9043=CARTESIAN_POINT('Ctrl Pts',(93.8044,2.9949745652833,-2.25101597516272));
#9044=CARTESIAN_POINT('Ctrl Pts',(93.8044,2.98510962519026,-2.26638162179989));
#9045=CARTESIAN_POINT('Ctrl Pts',(93.8044,2.98022249157794,-2.27399382901528));
#9046=CARTESIAN_POINT('Ctrl Pts',(93.8044,2.97530477836654,-2.28158703606508));
#9047=CARTESIAN_POINT('Ctrl Pts',(93.8044,2.97035813611545,-2.28915855262409));
#9048=CARTESIAN_POINT('Ctrl Pts',(93.8044,2.9087203455497,-2.38350367164438));
#9049=CARTESIAN_POINT('Ctrl Pts',(93.8044,2.84252153743242,-2.47459708052516));
#9050=CARTESIAN_POINT('Ctrl Pts',(93.8044,2.77218312951852,-2.56235147997252));
#9051=CARTESIAN_POINT('Ctrl Pts',(93.8044,2.69908607066416,-2.65354758024516));
#9052=CARTESIAN_POINT('Ctrl Pts',(93.8044,2.62151807644388,-2.74113813397251));
#9053=CARTESIAN_POINT('Ctrl Pts',(93.8044,2.53989902016449,-2.82500568909054));
#9054=CARTESIAN_POINT('Ctrl Pts',(93.8044,2.4567843214,-2.91041008969875));
#9055=CARTESIAN_POINT('Ctrl Pts',(93.8044,2.36946820531788,-2.99195432509609));
#9056=CARTESIAN_POINT('Ctrl Pts',(93.8044,2.27834636313374,-3.06948664813827));
#9057=CARTESIAN_POINT('Ctrl Pts',(93.8044,2.21740536476488,-3.12133916844289));
#9058=CARTESIAN_POINT('Ctrl Pts',(93.8044,2.15476118149509,-3.17139668069635));
#9059=CARTESIAN_POINT('Ctrl Pts',(93.8044,2.09052247727841,-3.21960525239369));
#9060=CARTESIAN_POINT('Ctrl Pts',(93.8044,2.06033097035291,-3.24226276773458));
#9061=CARTESIAN_POINT('Ctrl Pts',(93.8044,2.02978714981905,-3.26451176450614));
#9062=CARTESIAN_POINT('Ctrl Pts',(93.8044,1.99890180904653,-3.28634604859549));
#9063=CARTESIAN_POINT('Ctrl Pts',(93.8044,1.98422286547466,-3.29672327662868));
#9064=CARTESIAN_POINT('Ctrl Pts',(93.8044,1.96946536617489,-3.30700778786405));
#9065=CARTESIAN_POINT('Ctrl Pts',(93.8044,1.95463485827397,-3.31719585920331));
#9066=CARTESIAN_POINT('Ctrl Pts',(93.8044,1.84995490991091,-3.38910754212328));
#9067=CARTESIAN_POINT('Ctrl Pts',(93.8044,1.74200124640053,-3.45597177584477));
#9068=CARTESIAN_POINT('Ctrl Pts',(93.8044,1.63126903045248,-3.51765019114321));
#9069=CARTESIAN_POINT('Ctrl Pts',(93.8044,1.52297675373357,-3.57796954770892));
#9070=CARTESIAN_POINT('Ctrl Pts',(93.8044,1.41202606433326,-3.63332946958868));
#9071=CARTESIAN_POINT('Ctrl Pts',(93.8044,1.298836561106,-3.68356636248008));
#9072=CARTESIAN_POINT('Ctrl Pts',(93.8044,1.18182163951623,-3.73550109065712));
#9073=CARTESIAN_POINT('Ctrl Pts',(93.8044,1.0624133428104,-3.78196146339442));
#9074=CARTESIAN_POINT('Ctrl Pts',(93.8044,0.941040083796187,-3.82272044533804));
#9075=CARTESIAN_POINT('Ctrl Pts',(93.8044,0.819666824781972,-3.86347942728167));
#9076=CARTESIAN_POINT('Ctrl Pts',(93.8044,0.696327677346945,-3.8985376289676));
#9077=CARTESIAN_POINT('Ctrl Pts',(93.8044,0.571428919000175,-3.92761210585552));
#9078=CARTESIAN_POINT('Ctrl Pts',(93.8044,-2.97061198327651,-2.63181325464289));
#9079=CARTESIAN_POINT('Ctrl Pts',(93.8044,-3.04430299923343,-2.53520263969804));
#9080=CARTESIAN_POINT('Ctrl Pts',(93.8044,-3.11302395750424,-2.43516079500702));
#9081=CARTESIAN_POINT('Ctrl Pts',(93.8044,-3.17676704501544,-2.33211195540638));
#9082=CARTESIAN_POINT('Ctrl Pts',(93.8044,-3.24169167615227,-2.22715299967689));
#9083=CARTESIAN_POINT('Ctrl Pts',(93.8044,-3.30145240555427,-2.11907371594739));
#9084=CARTESIAN_POINT('Ctrl Pts',(93.8044,-3.3559920719374,-2.00829996844531));
#9085=CARTESIAN_POINT('Ctrl Pts',(93.8044,-3.41270540168603,-1.89311136378014));
#9086=CARTESIAN_POINT('Ctrl Pts',(93.8044,-3.46377367315599,-1.7750082788633));
#9087=CARTESIAN_POINT('Ctrl Pts',(93.8044,-3.50907466073431,-1.6544593061801));
#9088=CARTESIAN_POINT('Ctrl Pts',(93.8044,-3.51614057890727,-1.63565642301245));
#9089=CARTESIAN_POINT('Ctrl Pts',(93.8044,-3.52306606694267,-1.61679403209505));
#9090=CARTESIAN_POINT('Ctrl Pts',(93.8044,-3.52985052887756,-1.5978739149434));
#9091=CARTESIAN_POINT('Ctrl Pts',(93.8044,-3.53663923027215,-1.57894197503045));
#9092=CARTESIAN_POINT('Ctrl Pts',(93.8044,-3.54328414598354,-1.55995934744993));
#9093=CARTESIAN_POINT('Ctrl Pts',(93.8044,-3.5497830310177,-1.54093389587887));
#9094=CARTESIAN_POINT('Ctrl Pts',(93.8044,-3.58935229555709,-1.42509508318412));
#9095=CARTESIAN_POINT('Ctrl Pts',(93.8044,-3.62353728821377,-1.30759982045371));
#9096=CARTESIAN_POINT('Ctrl Pts',(93.8044,-3.65228644268449,-1.18886601820872));
#9097=CARTESIAN_POINT('Ctrl Pts',(93.8044,-3.68089336281439,-1.07071964277349));
#9098=CARTESIAN_POINT('Ctrl Pts',(93.8044,-3.70411811636173,-0.951346066625019));
#9099=CARTESIAN_POINT('Ctrl Pts',(93.8044,-3.72185879396385,-0.831153747601256));
#9100=CARTESIAN_POINT('Ctrl Pts',(93.8044,-3.73309728149118,-0.755013483484906));
#9101=CARTESIAN_POINT('Ctrl Pts',(93.8044,-3.74213395530222,-0.678544631812329));
#9102=CARTESIAN_POINT('Ctrl Pts',(93.8044,-3.74893214499955,-0.601852766463008));
#9103=CARTESIAN_POINT('Ctrl Pts',(93.8044,-3.75249425141003,-0.561667864694248));
#9104=CARTESIAN_POINT('Ctrl Pts',(93.8044,-3.75544163433645,-0.521421767935013));
#9105=CARTESIAN_POINT('Ctrl Pts',(93.8044,-3.75776809086273,-0.481129960395163));
#9106=CARTESIAN_POINT('Ctrl Pts',(93.8044,-3.75893451047219,-0.46092878582595));
#9107=CARTESIAN_POINT('Ctrl Pts',(93.8044,-3.75994480481882,-0.440714836914725));
#9108=CARTESIAN_POINT('Ctrl Pts',(93.8044,-3.76079753130694,-0.420510350725053));
#9109=CARTESIAN_POINT('Ctrl Pts',(93.8044,-3.76583949284932,-0.301046203930483));
#9110=CARTESIAN_POINT('Ctrl Pts',(93.8044,-3.76538761743502,-0.181748933042815));
#9111=CARTESIAN_POINT('Ctrl Pts',(93.8044,-3.75937625299169,-0.06300757537429));
#9112=CARTESIAN_POINT('Ctrl Pts',(93.8044,-3.75347847998659,0.0534900318575171));
#9113=CARTESIAN_POINT('Ctrl Pts',(93.8044,-3.74222921402806,0.169453309647518));
#9114=CARTESIAN_POINT('Ctrl Pts',(93.8044,-3.72551718295993,0.284506526530065));
#9115=CARTESIAN_POINT('Ctrl Pts',(93.8044,-3.70832233991097,0.402883640509215));
#9116=CARTESIAN_POINT('Ctrl Pts',(93.8044,-3.68534483519235,0.520298295770664));
#9117=CARTESIAN_POINT('Ctrl Pts',(93.8044,-3.65640891355301,0.6363191991641));
#9118=CARTESIAN_POINT('Ctrl Pts',(93.8044,-3.64194095273334,0.694329650860818));
#9119=CARTESIAN_POINT('Ctrl Pts',(93.8044,-3.62598251867022,0.751991234600619));
#9120=CARTESIAN_POINT('Ctrl Pts',(93.8044,-3.60850639143369,0.809246906377294));
#9121=CARTESIAN_POINT('Ctrl Pts',(93.8044,-3.59937124006994,0.83917568985628));
#9122=CARTESIAN_POINT('Ctrl Pts',(93.8044,-3.58982133903167,0.868993523663466));
#9123=CARTESIAN_POINT('Ctrl Pts',(93.8044,-3.57985241638791,0.898691981790592));
#9124=CARTESIAN_POINT('Ctrl Pts',(93.8044,-3.57385050346129,0.916572305081645));
#9125=CARTESIAN_POINT('Ctrl Pts',(93.8044,-3.56769669888428,0.934409353348099));
#9126=CARTESIAN_POINT('Ctrl Pts',(93.8044,-3.56139002402582,0.952201251079662));
#9127=CARTESIAN_POINT('Ctrl Pts',(93.8044,-3.55813224683699,0.961391837224778));
#9128=CARTESIAN_POINT('Ctrl Pts',(93.8044,-3.55483353387343,0.970570734195694));
#9129=CARTESIAN_POINT('Ctrl Pts',(93.8044,-3.55149565259232,0.979732558860926));
#9130=CARTESIAN_POINT('Ctrl Pts',(93.8044,-3.51235991575605,1.08715242459066));
#9131=CARTESIAN_POINT('Ctrl Pts',(93.8044,-3.46778751151284,1.19238879397286));
#9132=CARTESIAN_POINT('Ctrl Pts',(93.8044,-3.41814899903905,1.29519935184003));
#9133=CARTESIAN_POINT('Ctrl Pts',(93.8044,-3.36777050532375,1.39954254798461));
#9134=CARTESIAN_POINT('Ctrl Pts',(93.8044,-3.31217307851915,1.50138772187045));
#9135=CARTESIAN_POINT('Ctrl Pts',(93.8044,-3.25169578138477,1.60045450315049));
#9136=CARTESIAN_POINT('Ctrl Pts',(93.8044,-3.19103541880398,1.69982116067168));
#9137=CARTESIAN_POINT('Ctrl Pts',(93.8044,-3.12546484916859,1.79639319701438));
#9138=CARTESIAN_POINT('Ctrl Pts',(93.8044,-3.0552887223657,1.88985113911308));
#9139=CARTESIAN_POINT('Ctrl Pts',(93.8044,-3.01248668863769,1.94685328745185));
#9140=CARTESIAN_POINT('Ctrl Pts',(93.8044,-2.96797067855792,2.00269622303262));
#9141=CARTESIAN_POINT('Ctrl Pts',(93.8044,-2.92180480031303,2.05729932119145));
#9142=CARTESIAN_POINT('Ctrl Pts',(93.8044,-2.8974752368903,2.08607532611623));
#9143=CARTESIAN_POINT('Ctrl Pts',(93.8044,-2.87268739712321,2.11450687795852));
#9144=CARTESIAN_POINT('Ctrl Pts',(93.8044,-2.84745035132856,2.14258139753));
#9145=CARTESIAN_POINT('Ctrl Pts',(93.8044,-2.83607676292311,2.15523375125178));
#9146=CARTESIAN_POINT('Ctrl Pts',(93.8044,-2.82461122656622,2.16781425815774));
#9147=CARTESIAN_POINT('Ctrl Pts',(93.8044,-2.8130660969007,2.18030952282467));
#9148=CARTESIAN_POINT('Ctrl Pts',(93.8044,-2.73519313430374,2.26459123348869));
#9149=CARTESIAN_POINT('Ctrl Pts',(93.8044,-2.65358357547324,2.34513111386511));
#9150=CARTESIAN_POINT('Ctrl Pts',(93.8044,-2.56856063424907,2.42166304210725));
#9151=CARTESIAN_POINT('Ctrl Pts',(93.8044,-2.48400757560809,2.49777201367885));
#9152=CARTESIAN_POINT('Ctrl Pts',(93.8044,-2.39607798172114,2.56991771912839));
#9153=CARTESIAN_POINT('Ctrl Pts',(93.8044,-2.30506019564923,2.63779669698566));
#9154=CARTESIAN_POINT('Ctrl Pts',(93.8044,-2.21644895728947,2.70388092674022));
#9155=CARTESIAN_POINT('Ctrl Pts',(93.8044,-2.12490994173969,2.76592135953484));
#9156=CARTESIAN_POINT('Ctrl Pts',(93.8044,-2.03069231632377,2.82359275721866));
#9157=CARTESIAN_POINT('Ctrl Pts',(93.8044,-1.94022059772342,2.87897125396497));
#9158=CARTESIAN_POINT('Ctrl Pts',(93.8044,-1.84727844616327,2.9303213184372));
#9159=CARTESIAN_POINT('Ctrl Pts',(93.8044,-1.75208009336914,2.97731016051328));
#9160=CARTESIAN_POINT('Origin',(73.0447820522122,0.,0.));
#9161=CARTESIAN_POINT('Ctrl Pts',(75.6906153855455,-3.97203085734017,-0.00290119714995075));
#9162=CARTESIAN_POINT('Ctrl Pts',(75.6989285376769,-3.97366559007733,-0.198262094710035));
#9163=CARTESIAN_POINT('Ctrl Pts',(75.7630714588146,-3.87194711440902,-1.70397919582139));
#9164=CARTESIAN_POINT('Ctrl Pts',(75.8830441489587,-1.9464585018686,-4.26281795947025));
#9165=CARTESIAN_POINT('Ctrl Pts',(76.0505334559777,2.51279058774102,-3.9549296545997));
#9166=CARTESIAN_POINT('Ctrl Pts',(76.2180227629969,4.68558178106048,-0.0490381362345196));
#9167=CARTESIAN_POINT('Ctrl Pts',(76.3855120700159,2.59485425351327,3.90182050286693));
#9168=CARTESIAN_POINT('Ctrl Pts',(76.553001377035,-1.85699592939576,4.30214329460675));
#9169=CARTESIAN_POINT('Ctrl Pts',(76.674146926656,-3.85484883176064,1.76030277155817));
#9170=CARTESIAN_POINT('Ctrl Pts',(76.7394627072706,-3.97321680284677,0.22630718179755));
#9171=CARTESIAN_POINT('Ctrl Pts',(76.7489487188789,-3.97125648760866,0.00321799934434826));
#9172=CARTESIAN_POINT('Ctrl Pts',(75.5236667307631,-3.97344267433394,0.0030056548558996));
#9173=CARTESIAN_POINT('Ctrl Pts',(75.5749566001284,-3.96619874465367,-1.19966076974019));
#9174=CARTESIAN_POINT('Ctrl Pts',(75.6820762385001,-2.74440924139197,-3.73144021430678));
#9175=CARTESIAN_POINT('Ctrl Pts',(75.8450256458783,1.55028466462108,-4.42080615645044));
#9176=CARTESIAN_POINT('Ctrl Pts',(76.0125149528972,4.55194904417391,-1.11163115411373));
#9177=CARTESIAN_POINT('Ctrl Pts',(76.1800042599164,3.41272104871659,3.21148763121955));
#9178=CARTESIAN_POINT('Ctrl Pts',(76.3474935669354,-0.83234909652074,4.61115832194601));
#9179=CARTESIAN_POINT('Ctrl Pts',(76.4814921683288,-3.62244148753537,2.37463487493447));
#9180=CARTESIAN_POINT('Ctrl Pts',(76.5596610007158,-3.96584760293371,0.530055364675002));
#9181=CARTESIAN_POINT('Ctrl Pts',(76.5820000640964,-3.96340732379332,0.00203673152180048));
#9182=CARTESIAN_POINT('Ctrl Pts',(75.342557724821,2.66903922910596,-2.1929680694195));
#9183=CARTESIAN_POINT('Ctrl Pts',(75.3983874938273,3.3959072005702,-1.30830442234129));
#9184=CARTESIAN_POINT('Ctrl Pts',(75.5100470318401,3.88844938254442,1.22557529574225));
#9185=CARTESIAN_POINT('Ctrl Pts',(75.6775363388591,1.08737198548797,3.93348015258173));
#9186=CARTESIAN_POINT('Ctrl Pts',(75.8450256458782,-2.70311334847693,3.05287906662549));
#9187=CARTESIAN_POINT('Ctrl Pts',(76.0125149528973,-4.03392091718051,-0.601029078824585));
#9188=CARTESIAN_POINT('Ctrl Pts',(76.1800042599164,-1.69419748002643,-3.71035675192291));
#9189=CARTESIAN_POINT('Ctrl Pts',(76.3474935669354,2.18713292756978,-3.44237077136358));
#9190=CARTESIAN_POINT('Ctrl Pts',(76.5149828739546,4.07833038223504,-0.0426827937785228));
#9191=CARTESIAN_POINT('Ctrl Pts',(76.6824721809735,2.25856114225795,3.39614456569537));
#9192=CARTESIAN_POINT('Ctrl Pts',(76.8499614879927,-1.61632925694607,3.74458552362572));
#9193=CARTESIAN_POINT('Ctrl Pts',(77.0174507950117,-4.02048175693465,0.685815660826552));
#9194=CARTESIAN_POINT('Ctrl Pts',(77.1849401020308,-2.76630182357442,-2.99703369017865));
#9195=CARTESIAN_POINT('Ctrl Pts',(77.3524294090499,1.00500289411644,-3.95279010425736));
#9196=CARTESIAN_POINT('Ctrl Pts',(77.519918716069,3.86183118677738,-1.31181793073376));
#9197=CARTESIAN_POINT('Ctrl Pts',(77.687408023088,3.20468654342747,2.52281404024267));
#9198=CARTESIAN_POINT('Ctrl Pts',(77.8548973301072,-0.36847943830367,4.06187428083153));
#9199=CARTESIAN_POINT('Ctrl Pts',(78.0223866371261,-3.60635710548903,1.90493881793867));
#9200=CARTESIAN_POINT('Ctrl Pts',(78.1898759441453,-3.5627237816556,-1.98534692649581));
#9201=CARTESIAN_POINT('Ctrl Pts',(78.3573652511643,-0.277282462911693,-4.06911744938491));
#9202=CARTESIAN_POINT('Ctrl Pts',(78.5248545581834,3.26046483027065,-2.45030038641864));
#9203=CARTESIAN_POINT('Ctrl Pts',(78.6923438652025,3.83143681832768,1.39810397265408));
#9204=CARTESIAN_POINT('Ctrl Pts',(78.8598331722216,0.916092365606468,3.97433988259736));
#9205=CARTESIAN_POINT('Ctrl Pts',(79.0273224792407,-2.83282654630066,2.93422844240184));
#9206=CARTESIAN_POINT('Ctrl Pts',(79.1948117862598,-4.00408850385809,-0.775807985939492));
#9207=CARTESIAN_POINT('Ctrl Pts',(79.3623010932788,-1.53193410324385,-3.77991807743596));
#9208=CARTESIAN_POINT('Ctrl Pts',(79.5297904002979,2.33416395414478,-3.3445898721694));
#9209=CARTESIAN_POINT('Ctrl Pts',(79.697279707317,4.07635013378049,0.134061038278646));
#9210=CARTESIAN_POINT('Ctrl Pts',(79.8647690143361,2.10936736161653,3.49072658741202));
#9211=CARTESIAN_POINT('Ctrl Pts',(80.0322583213552,-1.77697946634019,3.67109612400433));
#9212=CARTESIAN_POINT('Ctrl Pts',(80.1997476283741,-4.04640997254009,0.51104707139247));
#9213=CARTESIAN_POINT('Ctrl Pts',(80.3672369353934,-2.63391479920022,-3.11401599314157));
#9214=CARTESIAN_POINT('Ctrl Pts',(80.5347262424123,1.17524274960356,-3.90556106784105));
#9215=CARTESIAN_POINT('Ctrl Pts',(80.7022155494315,3.91501867647076,-1.14334226631976));
#9216=CARTESIAN_POINT('Ctrl Pts',(80.8697048564505,3.0924250217599,2.65923114073586));
#9217=CARTESIAN_POINT('Ctrl Pts',(81.0371941634696,-0.544040479089439,4.04210622475407));
#9218=CARTESIAN_POINT('Ctrl Pts',(81.2046834704887,-3.6854704733388,1.74697171277105));
#9219=CARTESIAN_POINT('Ctrl Pts',(81.3721727775078,-3.47340231266724,-2.13777434483456));
#9220=CARTESIAN_POINT('Ctrl Pts',(81.5396620845269,-0.100801913007151,-4.07730814992086));
#9221=CARTESIAN_POINT('Ctrl Pts',(81.7071513915459,3.36352056982451,-2.30680128130774));
#9222=CARTESIAN_POINT('Ctrl Pts',(81.874640698565,3.76729485221803,1.56271951146948));
#9223=CARTESIAN_POINT('Ctrl Pts',(82.0421300055841,0.743117010900478,4.01028426463592));
#9224=CARTESIAN_POINT('Ctrl Pts',(82.2096193126031,-2.9572408576274,2.80879498807853));
#9225=CARTESIAN_POINT('Ctrl Pts',(82.3771086196223,-3.96673419978018,-0.948484350619567));
#9226=CARTESIAN_POINT('Ctrl Pts',(82.5445979266412,-1.36680076284027,-3.8427149841974));
#9227=CARTESIAN_POINT('Ctrl Pts',(82.7120872336604,2.47681753590696,-3.24036690343852));
#9228=CARTESIAN_POINT('Ctrl Pts',(82.8795765406795,4.06672003450697,0.310468897018032));
#9229=CARTESIAN_POINT('Ctrl Pts',(83.0470658476984,1.95621624008245,3.57880158672057));
#9230=CARTESIAN_POINT('Ctrl Pts',(83.2145551547178,-1.93429572404523,3.5906967049608));
#9231=CARTESIAN_POINT('Ctrl Pts',(83.3820444617366,-4.06474552281777,0.335330597781985));
#9232=CARTESIAN_POINT('Ctrl Pts',(83.5495337687559,-2.49658568420434,-3.22516087916586));
#9233=CARTESIAN_POINT('Ctrl Pts',(83.7170230757748,1.343277467771,-3.85100096334118));
#9234=CARTESIAN_POINT('Ctrl Pts',(83.8845123827939,3.96086016944716,-0.9727227216237));
#9235=CARTESIAN_POINT('Ctrl Pts',(84.052001689813,2.97436101339852,2.79065930150043));
#9236=CARTESIAN_POINT('Ctrl Pts',(84.219490996832,-0.718580710202222,4.0147533595479));
#9237=CARTESIAN_POINT('Ctrl Pts',(84.3869803038512,-3.75766857626771,1.5857268510075));
#9238=CARTESIAN_POINT('Ctrl Pts',(84.5544696108703,-3.37756349845322,-2.28619062831437));
#9239=CARTESIAN_POINT('Ctrl Pts',(84.7219589178894,0.0758677780459848,-4.07784831195696));
#9240=CARTESIAN_POINT('Ctrl Pts',(84.8894482249084,3.46026514000546,-2.15897381548248));
#9241=CARTESIAN_POINT('Ctrl Pts',(85.0569375319275,3.69608409210104,1.72440284133193));
#9242=CARTESIAN_POINT('Ctrl Pts',(85.2244268389465,0.568747302491688,4.0387039110319));
#9243=CARTESIAN_POINT('Ctrl Pts',(85.3919161459657,-3.0761063260992,2.67809123175602));
#9244=CARTESIAN_POINT('Ctrl Pts',(85.5594054529847,-3.92193688191295,-1.11938102063903));
#9245=CARTESIAN_POINT('Ctrl Pts',(85.7268947600039,-1.19910281475489,-3.89830158078141));
#9246=CARTESIAN_POINT('Ctrl Pts',(85.8943840670228,2.61482372103935,-3.13006384646798));
#9247=CARTESIAN_POINT('Ctrl Pts',(86.061873374042,4.04945931219474,0.486294205142611));
#9248=CARTESIAN_POINT('Ctrl Pts',(86.229362681061,1.79939455637655,3.66016147260723));
#9249=CARTESIAN_POINT('Ctrl Pts',(86.3968519880802,-2.08798255031681,3.50355985315628));
#9250=CARTESIAN_POINT('Ctrl Pts',(86.5643412950992,-4.07545415494521,0.158984923863421));
#9251=CARTESIAN_POINT('Ctrl Pts',(86.7318306021182,-2.35457208045918,-3.33025420846489));
#9252=CARTESIAN_POINT('Ctrl Pts',(86.8993199091373,1.50879171639289,-3.78921500203144));
#9253=CARTESIAN_POINT('Ctrl Pts',(87.0668092161565,3.99926967039633,-0.800278000774745));
#9254=CARTESIAN_POINT('Ctrl Pts',(87.2342985231755,2.85071603868332,2.91685118610285));
#9255=CARTESIAN_POINT('Ctrl Pts',(87.4017878301946,-0.891772626585205,3.9798673793921));
#9256=CARTESIAN_POINT('Ctrl Pts',(87.5692771372136,-3.8228159473593,1.42150659783601));
#9257=CARTESIAN_POINT('Ctrl Pts',(87.7367664442328,-3.27538716564014,-2.43031719951029));
#9258=CARTESIAN_POINT('Ctrl Pts',(87.9042557512518,0.252395113979941,-4.07073697031827));
#9259=CARTESIAN_POINT('Ctrl Pts',(88.0717450582709,3.55051701369304,-2.00709534166942));
#9260=CARTESIAN_POINT('Ctrl Pts',(88.23923436529,3.6179381546919,1.88285057396995));
#9261=CARTESIAN_POINT('Ctrl Pts',(88.406723672309,0.393310420479956,4.05954550266719));
#9262=CARTESIAN_POINT('Ctrl Pts',(88.5742129793281,-3.18919991757636,2.54236241727983));
#9263=CARTESIAN_POINT('Ctrl Pts',(88.7417022863473,-3.86978060604414,-1.2881773310196));
#9264=CARTESIAN_POINT('Ctrl Pts',(88.9091915933662,-1.02915492040045,-3.94657356765929));
#9265=CARTESIAN_POINT('Ctrl Pts',(89.0766809003854,2.74792356052482,-3.01388766885894));
#9266=CARTESIAN_POINT('Ctrl Pts',(89.2441702074045,4.02460035413828,0.661207051172942));
#9267=CARTESIAN_POINT('Ctrl Pts',(89.4116595144235,1.63919656413269,3.73465358495402));
#9268=CARTESIAN_POINT('Ctrl Pts',(89.5791488214426,-2.23775157363024,3.40984906836557));
#9269=CARTESIAN_POINT('Ctrl Pts',(89.7466381284617,-4.07851577570426,-0.0176590624915208));
#9270=CARTESIAN_POINT('Ctrl Pts',(89.9141274354808,-2.20814045631811,-3.42909878875167));
#9271=CARTESIAN_POINT('Ctrl Pts',(90.0816167424998,1.67147493142775,-3.72031911566969));
#9272=CARTESIAN_POINT('Ctrl Pts',(90.2491060495189,4.03017510942306,-0.626331673446937));
#9273=CARTESIAN_POINT('Ctrl Pts',(90.4165953565381,2.72172209969999,3.03757001658075));
#9274=CARTESIAN_POINT('Ctrl Pts',(90.584084663557,-1.06329125786327,3.93751373657007));
#9275=CARTESIAN_POINT('Ctrl Pts',(90.7515739705761,-3.88079034745029,1.25461910168971));
#9276=CARTESIAN_POINT('Ctrl Pts',(90.9190632775953,-3.16706503236784,-2.5698836498698));
#9277=CARTESIAN_POINT('Ctrl Pts',(91.0865525846142,0.428448863837588,-4.05598742012391));
#9278=CARTESIAN_POINT('Ctrl Pts',(91.2540418916334,3.63410685090686,-1.85145093348772));
#9279=CARTESIAN_POINT('Ctrl Pts',(91.4215311986524,3.53300366018645,2.03776559238545));
#9280=CARTESIAN_POINT('Ctrl Pts',(91.5890205056715,0.217135566134788,4.07276956328891));
#9281=CARTESIAN_POINT('Ctrl Pts',(91.7565098126906,-3.29630946515284,2.401863949772));
#9282=CARTESIAN_POINT('Ctrl Pts',(91.9239991197097,-3.81036316275665,-1.45455799694203));
#9283=CARTESIAN_POINT('Ctrl Pts',(92.0914884267288,-0.85727610730619,-3.98743753572885));
#9284=CARTESIAN_POINT('Ctrl Pts',(92.2589777337478,2.87586759608463,-2.89206194417883));
#9285=CARTESIAN_POINT('Ctrl Pts',(92.426467040767,3.99218924348707,0.834890245879901));
#9286=CARTESIAN_POINT('Ctrl Pts',(92.593956347786,1.4759239582885,3.80211644744834));
#9287=CARTESIAN_POINT('Ctrl Pts',(92.7614456548051,-2.38332395405469,3.30978296485569));
#9288=CARTESIAN_POINT('Ctrl Pts',(92.9289349618241,-4.07392034251622,-0.194354239414968));
#9289=CARTESIAN_POINT('Ctrl Pts',(93.0964242688434,-2.05757404133894,-3.52134293058862));
#9290=CARTESIAN_POINT('Ctrl Pts',(93.2639135758622,1.8310385540054,-3.64477024538087));
#9291=CARTESIAN_POINT('Ctrl Pts',(93.4314028828815,4.05348565523183,-0.450564049263689));
#9292=CARTESIAN_POINT('Ctrl Pts',(93.5988921899005,2.58768524108504,3.15131360915174));
#9293=CARTESIAN_POINT('Ctrl Pts',(93.7663814969195,-1.23293249244653,3.89031122336608));
#9294=CARTESIAN_POINT('Ctrl Pts',(93.9338708039387,-3.93134593579687,1.0800891348575));
#9295=CARTESIAN_POINT('Ctrl Pts',(94.0455303419513,-3.34489230679012,-1.43371602222286));
#9296=CARTESIAN_POINT('Ctrl Pts',(94.1013601109577,-2.58562067024381,-2.29073025684125));
#9297=CARTESIAN_POINT('Ctrl Pts',(75.2435710211684,2.80150992613879,-2.30181023462966));
#9298=CARTESIAN_POINT('Ctrl Pts',(75.2994007901748,3.56445406530438,-1.37323864918543));
#9299=CARTESIAN_POINT('Ctrl Pts',(75.4110603281875,4.08144227469277,1.28640348137652));
#9300=CARTESIAN_POINT('Ctrl Pts',(75.5785496352065,1.14134081565006,4.12870802780178));
#9301=CARTESIAN_POINT('Ctrl Pts',(75.7460389422257,-2.83727522422854,3.20440063794697));
#9302=CARTESIAN_POINT('Ctrl Pts',(75.9135282492446,-4.23413390387881,-0.630859566192717));
#9303=CARTESIAN_POINT('Ctrl Pts',(76.0810175562638,-1.77828448730715,-3.89451048777202));
#9304=CARTESIAN_POINT('Ctrl Pts',(76.2485068632828,2.29568548096019,-3.61322373244229));
#9305=CARTESIAN_POINT('Ctrl Pts',(76.415996170302,4.28074751517686,-0.0448012412638526));
#9306=CARTESIAN_POINT('Ctrl Pts',(76.583485477321,2.37065884600972,3.56470321141922));
#9307=CARTESIAN_POINT('Ctrl Pts',(76.7509747843401,-1.69655148109597,3.93043811395273));
#9308=CARTESIAN_POINT('Ctrl Pts',(76.9184640913592,-4.22002772648839,0.719854305757281));
#9309=CARTESIAN_POINT('Ctrl Pts',(77.0859533983782,-2.90359989202388,-3.14578352406619));
#9310=CARTESIAN_POINT('Ctrl Pts',(77.2534427053974,1.05488355246413,-4.14897637781425));
#9311=CARTESIAN_POINT('Ctrl Pts',(77.4209320124163,4.05350295523876,-1.3769265412665));
#9312=CARTESIAN_POINT('Ctrl Pts',(77.5884213194355,3.3637426770167,2.64802723709294));
#9313=CARTESIAN_POINT('Ctrl Pts',(77.7559106264545,-0.386767939837125,4.26347465874045));
#9314=CARTESIAN_POINT('Ctrl Pts',(77.9233999334736,-3.78534909418059,1.99948541368194));
#9315=CARTESIAN_POINT('Ctrl Pts',(78.0908892404927,-3.73955014581866,-2.08388436586233));
#9316=CARTESIAN_POINT('Ctrl Pts',(78.2583785475118,-0.291044643975323,-4.27107732279188));
#9317=CARTESIAN_POINT('Ctrl Pts',(78.4258678545309,3.42228937147894,-2.57191456000927));
#9318=CARTESIAN_POINT('Ctrl Pts',(78.59335716155,4.02160004276674,1.46749516247331));
#9319=CARTESIAN_POINT('Ctrl Pts',(78.760846468569,0.961560185222965,4.17159572235863));
#9320=CARTESIAN_POINT('Ctrl Pts',(78.9283357755881,-2.97342639326778,3.07986110406517));
#9321=CARTESIAN_POINT('Ctrl Pts',(79.0958250826072,-4.20282083768928,-0.814313161712223));
#9322=CARTESIAN_POINT('Ctrl Pts',(79.2633143896262,-1.60796759733868,-3.967524305544));
#9323=CARTESIAN_POINT('Ctrl Pts',(79.4308036966454,2.45001400333946,-3.5105897371484));
#9324=CARTESIAN_POINT('Ctrl Pts',(79.5982930036644,4.27866898233209,0.140714803046155));
#9325=CARTESIAN_POINT('Ctrl Pts',(79.7657823106835,2.21406022699088,3.6639795614196));
#9326=CARTESIAN_POINT('Ctrl Pts',(79.9332716177026,-1.86517513838281,3.8533012625119));
#9327=CARTESIAN_POINT('Ctrl Pts',(80.1007609247216,-4.24724282044189,0.536411540009373));
#9328=CARTESIAN_POINT('Ctrl Pts',(80.2682502317408,-2.76464218813111,-3.26857193397764));
#9329=CARTESIAN_POINT('Ctrl Pts',(80.4357395387598,1.23357281254345,-4.09940325319346));
#9330=CARTESIAN_POINT('Ctrl Pts',(80.6032288457789,4.10933026519265,-1.20008903321431));
#9331=CARTESIAN_POINT('Ctrl Pts',(80.770718152798,3.24590935188401,2.79121503926503));
#9332=CARTESIAN_POINT('Ctrl Pts',(80.938207459817,-0.571042488161895,4.24272546752679));
#9333=CARTESIAN_POINT('Ctrl Pts',(81.1056967668361,-3.86838904462584,1.83367802939756));
#9334=CARTESIAN_POINT('Ctrl Pts',(81.2731860738552,-3.64579544215624,-2.24387711562598));
#9335=CARTESIAN_POINT('Ctrl Pts',(81.4406753808743,-0.105804949130666,-4.27967454706767));
#9336=CARTESIAN_POINT('Ctrl Pts',(81.6081646878933,3.53046000987095,-2.42129325666677));
#9337=CARTESIAN_POINT('Ctrl Pts',(81.7756539949125,3.95427455995679,1.6402809578108));
#9338=CARTESIAN_POINT('Ctrl Pts',(81.9431433019315,0.779999656662083,4.20932410865277));
#9339=CARTESIAN_POINT('Ctrl Pts',(82.1106326089506,-3.10401567960523,2.94820209226625));
#9340=CARTESIAN_POINT('Ctrl Pts',(82.2781219159697,-4.16361255160751,-0.995559860668701));
#9341=CARTESIAN_POINT('Ctrl Pts',(82.4456112229887,-1.43463830070183,-4.03343797054543));
#9342=CARTESIAN_POINT('Ctrl Pts',(82.6131005300079,2.59974781801999,-3.40119393724889));
#9343=CARTESIAN_POINT('Ctrl Pts',(82.7805898370269,4.26856091857257,0.325878198892089));
#9344=CARTESIAN_POINT('Ctrl Pts',(82.9480791440459,2.05330785493948,3.75642593017913));
#9345=CARTESIAN_POINT('Ctrl Pts',(83.1155684510651,-2.03029937211365,3.76891143112613));
#9346=CARTESIAN_POINT('Ctrl Pts',(83.2830577580841,-4.26648840722233,0.351973844363078));
#9347=CARTESIAN_POINT('Ctrl Pts',(83.4505470651033,-2.62049710603065,-3.3852332022127));
#9348=CARTESIAN_POINT('Ctrl Pts',(83.6180363721222,1.40994748914934,-4.04213520233054));
#9349=CARTESIAN_POINT('Ctrl Pts',(83.7855256791414,4.15744697932781,-1.02100123905723));
#9350=CARTESIAN_POINT('Ctrl Pts',(83.9530149861604,3.12198554899,2.92916628889107));
#9351=CARTESIAN_POINT('Ctrl Pts',(84.1205042931796,-0.754245561627699,4.21401501526076));
#9352=CARTESIAN_POINT('Ctrl Pts',(84.2879936001986,-3.944170509281,1.66443020574501));
#9353=CARTESIAN_POINT('Ctrl Pts',(84.4554829072177,-3.54519992208969,-2.39965964846967));
#9354=CARTESIAN_POINT('Ctrl Pts',(84.6229722142368,0.0796332743828251,-4.28024151861659));
#9355=CARTESIAN_POINT('Ctrl Pts',(84.7904615212558,3.63200624070426,-2.26612876588327));
#9356=CARTESIAN_POINT('Ctrl Pts',(84.957950828275,3.87952944226047,1.80998901176569));
#9357=CARTESIAN_POINT('Ctrl Pts',(85.125440135294,0.596975569343298,4.23915428896914));
#9358=CARTESIAN_POINT('Ctrl Pts',(85.2929294423131,-3.22878072096074,2.8110112009792));
#9359=CARTESIAN_POINT('Ctrl Pts',(85.4604187493321,-4.11659183744908,-1.17493853453105));
#9360=CARTESIAN_POINT('Ctrl Pts',(85.6279080563513,-1.25861710886957,-4.09178346070989));
#9361=CARTESIAN_POINT('Ctrl Pts',(85.7953973633703,2.74460357484093,-3.2854162800243));
#9362=CARTESIAN_POINT('Ctrl Pts',(85.9628866703894,4.25044350599852,0.510430130765498));
#9363=CARTESIAN_POINT('Ctrl Pts',(86.1303759774084,1.88870274207907,3.84182389863737));
#9364=CARTESIAN_POINT('Ctrl Pts',(86.2978652844277,-2.19161403718915,3.67744977233867));
#9365=CARTESIAN_POINT('Ctrl Pts',(86.4653545914466,-4.27772853395903,0.166875719716936));
#9366=CARTESIAN_POINT('Ctrl Pts',(86.6328438984657,-2.47143503298197,-3.49554256072326));
#9367=CARTESIAN_POINT('Ctrl Pts',(86.8003332054849,1.58367659937562,-3.97728265838227));
#9368=CARTESIAN_POINT('Ctrl Pts',(86.9678225125038,4.19776283418438,-0.839997680960255));
#9369=CARTESIAN_POINT('Ctrl Pts',(87.135311819523,2.99220378325032,3.0616213736484));
#9370=CARTESIAN_POINT('Ctrl Pts',(87.302801126542,-0.936033400331159,4.17739756182517));
#9371=CARTESIAN_POINT('Ctrl Pts',(87.4702904335611,-4.01255129768779,1.49205931500802));
#9372=CARTESIAN_POINT('Ctrl Pts',(87.6377797405801,-3.43795233746419,-2.5509395605154));
#9373=CARTESIAN_POINT('Ctrl Pts',(87.8052690475994,0.264922077357618,-4.2727772243598));
#9374=CARTESIAN_POINT('Ctrl Pts',(87.9727583546182,3.72673752724031,-2.10671220605374));
#9375=CARTESIAN_POINT('Ctrl Pts',(88.1402476616376,3.79750493810491,1.97630087819272));
#9376=CARTESIAN_POINT('Ctrl Pts',(88.3077369686564,0.412831342084664,4.26103029783633));
#9377=CARTESIAN_POINT('Ctrl Pts',(88.4752262756755,-3.34748741348548,2.66854584607865));
#9378=CARTESIAN_POINT('Ctrl Pts',(88.6427155826947,-4.06184692288824,-1.35211260296358));
#9379=CARTESIAN_POINT('Ctrl Pts',(88.8102048897137,-1.08023430064092,-4.14245129987768));
#9380=CARTESIAN_POINT('Ctrl Pts',(88.9776941967327,2.88430947253616,-3.1634740053648));
#9381=CARTESIAN_POINT('Ctrl Pts',(89.145183503752,4.22435073936205,0.694024312903952));
#9382=CARTESIAN_POINT('Ctrl Pts',(89.312672810771,1.72055374654368,3.92001322979548));
#9383=CARTESIAN_POINT('Ctrl Pts',(89.4801621177899,-2.34881644952734,3.57908790080283));
#9384=CARTESIAN_POINT('Ctrl Pts',(89.6476514248092,-4.28094211016017,-0.0185355233137089));
#9385=CARTESIAN_POINT('Ctrl Pts',(89.8151407318281,-2.31773566278978,-3.59929303010515));
#9386=CARTESIAN_POINT('Ctrl Pts',(89.9826300388472,1.7544341651567,-3.90496730707241));
#9387=CARTESIAN_POINT('Ctrl Pts',(90.1501193458664,4.23020218286869,-0.657417988121693));
#9388=CARTESIAN_POINT('Ctrl Pts',(90.3176086528855,2.8568075715601,3.18833176372722));
#9389=CARTESIAN_POINT('Ctrl Pts',(90.4850979599045,-1.11606490485281,4.13294180805425));
#9390=CARTESIAN_POINT('Ctrl Pts',(90.6525872669236,-4.07340310366565,1.31688879975151));
#9391=CARTESIAN_POINT('Ctrl Pts',(90.8200765739427,-3.32425392184198,-2.69743302219789));
#9392=CARTESIAN_POINT('Ctrl Pts',(90.9875658809617,0.449713789064823,-4.25729561928448));
#9393=CARTESIAN_POINT('Ctrl Pts',(91.1550551879808,3.81447612475701,-1.94334279967185));
#9394=CARTESIAN_POINT('Ctrl Pts',(91.3225444949999,3.70835494479128,2.13890469347811));
#9395=CARTESIAN_POINT('Ctrl Pts',(91.4900338020189,0.227912515189272,4.27491069970215));
#9396=CARTESIAN_POINT('Ctrl Pts',(91.6575231090381,-3.45991305993065,2.52107410904377));
#9397=CARTESIAN_POINT('Ctrl Pts',(91.8250124160571,-3.99948045208465,-1.52675113281967));
#9398=CARTESIAN_POINT('Ctrl Pts',(91.9925017230763,-0.899824737632048,-4.18534344283303));
#9399=CARTESIAN_POINT('Ctrl Pts',(92.1599910300952,3.0186036716256,-3.03560178332006));
#9400=CARTESIAN_POINT('Ctrl Pts',(92.3274803371144,4.19033098902778,0.87632781323056));
#9401=CARTESIAN_POINT('Ctrl Pts',(92.4949696441334,1.54917753710061,3.99082443289155));
#9402=CARTESIAN_POINT('Ctrl Pts',(92.6624589511525,-2.50161392971549,3.4740552811261));
#9403=CARTESIAN_POINT('Ctrl Pts',(92.8299482581716,-4.27611859481023,-0.204000497621225));
#9404=CARTESIAN_POINT('Ctrl Pts',(92.9974375651908,-2.15969628236128,-3.69611546574651));
#9405=CARTESIAN_POINT('Ctrl Pts',(93.1649268722097,1.9219173057667,-3.82566876858911));
#9406=CARTESIAN_POINT('Ctrl Pts',(93.3324161792289,4.25466968591429,-0.472926603179349));
#9407=CARTESIAN_POINT('Ctrl Pts',(93.4999054862479,2.71611814827125,3.30772071842949));
#9408=CARTESIAN_POINT('Ctrl Pts',(93.667394793267,-1.29412583306428,4.08339652305521));
#9409=CARTESIAN_POINT('Ctrl Pts',(93.834884100286,-4.1264678848162,1.13369650000667));
#9410=CARTESIAN_POINT('Ctrl Pts',(93.9465436382988,-3.51090718231095,-1.50487472185524));
#9411=CARTESIAN_POINT('Ctrl Pts',(94.0023734073051,-2.71395110792135,-2.40442458944182));
#9412=CARTESIAN_POINT('Ctrl Pts',(75.1445843175159,2.93398062317162,-2.41065239983982));
#9413=CARTESIAN_POINT('Ctrl Pts',(75.2004140865222,3.73300093003856,-1.43817287602958));
#9414=CARTESIAN_POINT('Ctrl Pts',(75.3120736245349,4.27443516684111,1.34723166701079));
#9415=CARTESIAN_POINT('Ctrl Pts',(75.479562931554,1.19530964581214,4.32393590302183));
#9416=CARTESIAN_POINT('Ctrl Pts',(75.6470522385732,-2.97143709998015,3.35592220926846));
#9417=CARTESIAN_POINT('Ctrl Pts',(75.8145415455921,-4.43434689057711,-0.66069005356085));
#9418=CARTESIAN_POINT('Ctrl Pts',(75.9820308526113,-1.86237149458788,-4.07866422362114));
#9419=CARTESIAN_POINT('Ctrl Pts',(76.1495201596303,2.40423803435061,-3.784076693521));
#9420=CARTESIAN_POINT('Ctrl Pts',(76.3170094666494,4.48316464811867,-0.0469196887491872));
#9421=CARTESIAN_POINT('Ctrl Pts',(76.4844987736684,2.4827565497615,3.73326185714308));
#9422=CARTESIAN_POINT('Ctrl Pts',(76.6519880806876,-1.77677370524587,4.11629070427974));
#9423=CARTESIAN_POINT('Ctrl Pts',(76.8194773877066,-4.41957369604213,0.753892950688012));
#9424=CARTESIAN_POINT('Ctrl Pts',(76.9869666947257,-3.04089796047335,-3.29453335795373));
#9425=CARTESIAN_POINT('Ctrl Pts',(77.1544560017448,1.10476421081183,-4.34516265137114));
#9426=CARTESIAN_POINT('Ctrl Pts',(77.3219453087638,4.24517472370013,-1.44203515179924));
#9427=CARTESIAN_POINT('Ctrl Pts',(77.4894346157829,3.52279881060593,2.77324043394322));
#9428=CARTESIAN_POINT('Ctrl Pts',(77.656923922802,-0.405056441370581,4.46507503664936));
#9429=CARTESIAN_POINT('Ctrl Pts',(77.8244132298211,-3.96434108287214,2.09403200942523));
#9430=CARTESIAN_POINT('Ctrl Pts',(77.9919025368402,-3.91637650998171,-2.18242180522885));
#9431=CARTESIAN_POINT('Ctrl Pts',(78.1593918438592,-0.304806825038957,-4.47303719619885));
#9432=CARTESIAN_POINT('Ctrl Pts',(78.3268811508783,3.58411391268723,-2.6935287335999));
#9433=CARTESIAN_POINT('Ctrl Pts',(78.4943704578975,4.21176326720579,1.53688635229255));
#9434=CARTESIAN_POINT('Ctrl Pts',(78.6618597649164,1.00702800483946,4.36885156211989));
#9435=CARTESIAN_POINT('Ctrl Pts',(78.8293490719356,-3.11402624023491,3.2254937657285));
#9436=CARTESIAN_POINT('Ctrl Pts',(78.9968383789546,-4.40155317152047,-0.852818337484957));
#9437=CARTESIAN_POINT('Ctrl Pts',(79.1643276859738,-1.6840010914335,-4.15513053365203));
#9438=CARTESIAN_POINT('Ctrl Pts',(79.3318169929927,2.56586405253415,-3.67658960212739));
#9439=CARTESIAN_POINT('Ctrl Pts',(79.4993063000118,4.4809878308837,0.14736856781366));
#9440=CARTESIAN_POINT('Ctrl Pts',(79.666795607031,2.31875309236523,3.83723253542718));
#9441=CARTESIAN_POINT('Ctrl Pts',(79.83428491405,-1.95337081042543,4.03550640101947));
#9442=CARTESIAN_POINT('Ctrl Pts',(80.0017742210691,-4.4480756683437,0.561776008626277));
#9443=CARTESIAN_POINT('Ctrl Pts',(80.1692635280882,-2.89536957706201,-3.42312787481371));
#9444=CARTESIAN_POINT('Ctrl Pts',(80.3367528351073,1.29190287548333,-4.29324543854586));
#9445=CARTESIAN_POINT('Ctrl Pts',(80.5042421421264,4.30364185391454,-1.25683580010885));
#9446=CARTESIAN_POINT('Ctrl Pts',(80.6717314491455,3.39939368200813,2.92319893779419));
#9447=CARTESIAN_POINT('Ctrl Pts',(80.8392207561645,-0.59804449723435,4.44334471029951));
#9448=CARTESIAN_POINT('Ctrl Pts',(81.0067100631835,-4.05130761591287,1.92038434602406));
#9449=CARTESIAN_POINT('Ctrl Pts',(81.1741993702027,-3.81818857164524,-2.3499798864174));
#9450=CARTESIAN_POINT('Ctrl Pts',(81.3416886772217,-0.110807985254183,-4.48204094421447));
#9451=CARTESIAN_POINT('Ctrl Pts',(81.5091779842408,3.69739944991738,-2.53578523202579));
#9452=CARTESIAN_POINT('Ctrl Pts',(81.6766672912599,4.14125426769555,1.71784240415212));
#9453=CARTESIAN_POINT('Ctrl Pts',(81.8441565982789,0.816882302423688,4.40836395266962));
#9454=CARTESIAN_POINT('Ctrl Pts',(82.0116459052981,-3.25079050158307,3.08760919645398));
#9455=CARTESIAN_POINT('Ctrl Pts',(82.1791352123171,-4.36049090343483,-1.04263537071784));
#9456=CARTESIAN_POINT('Ctrl Pts',(82.3466245193362,-1.50247583856339,-4.22416095689346));
#9457=CARTESIAN_POINT('Ctrl Pts',(82.5141138263553,2.72267810013302,-3.56202097105925));
#9458=CARTESIAN_POINT('Ctrl Pts',(82.6816031333744,4.47040180263817,0.341287500766147));
#9459=CARTESIAN_POINT('Ctrl Pts',(82.8490924403934,2.15039946979652,3.93405027363768));
#9460=CARTESIAN_POINT('Ctrl Pts',(83.0165817474126,-2.12630302018207,3.94712615729146));
#9461=CARTESIAN_POINT('Ctrl Pts',(83.1840710544315,-4.46823129162689,0.368617090944171));
#9462=CARTESIAN_POINT('Ctrl Pts',(83.3515603614508,-2.74440852785697,-3.54530552525954));
#9463=CARTESIAN_POINT('Ctrl Pts',(83.5190496684696,1.47661751052768,-4.2332694413199));
#9464=CARTESIAN_POINT('Ctrl Pts',(83.686538975489,4.35403378920846,-1.06927975649076));
#9465=CARTESIAN_POINT('Ctrl Pts',(83.8540282825078,3.26961008458147,3.06767327628172));
#9466=CARTESIAN_POINT('Ctrl Pts',(84.0215175895271,-0.789910413053178,4.41327667097361));
#9467=CARTESIAN_POINT('Ctrl Pts',(84.1890068965459,-4.13067244229429,1.74313356048251));
#9468=CARTESIAN_POINT('Ctrl Pts',(84.3564962035653,-3.71283634572615,-2.51312866862498));
#9469=CARTESIAN_POINT('Ctrl Pts',(84.523985510584,0.0833987707196642,-4.48263472527622));
#9470=CARTESIAN_POINT('Ctrl Pts',(84.6914748176035,3.80374734140306,-2.37328371628405));
#9471=CARTESIAN_POINT('Ctrl Pts',(84.8589641246222,4.06297479241989,1.89557518219944));
#9472=CARTESIAN_POINT('Ctrl Pts',(85.0264534316416,0.625203836194908,4.43960466690639));
#9473=CARTESIAN_POINT('Ctrl Pts',(85.1939427386604,-3.38145511582228,2.94393117020239));
#9474=CARTESIAN_POINT('Ctrl Pts',(85.3614320456797,-4.3112467929852,-1.23049604842306));
#9475=CARTESIAN_POINT('Ctrl Pts',(85.5289213526986,-1.31813140298424,-4.28526534063838));
#9476=CARTESIAN_POINT('Ctrl Pts',(85.6964106597178,2.87438342864251,-3.44076871358061));
#9477=CARTESIAN_POINT('Ctrl Pts',(85.8638999667368,4.45142769980231,0.534566056388386));
#9478=CARTESIAN_POINT('Ctrl Pts',(86.0313892737559,1.97801092778158,4.02348632466751));
#9479=CARTESIAN_POINT('Ctrl Pts',(86.198878580775,-2.29524552406149,3.85133969152105));
#9480=CARTESIAN_POINT('Ctrl Pts',(86.3663678877941,-4.48000291297286,0.174766515570451));
#9481=CARTESIAN_POINT('Ctrl Pts',(86.5338571948131,-2.58829798550476,-3.66083091298163));
#9482=CARTESIAN_POINT('Ctrl Pts',(86.7013465018322,1.65856148235836,-4.16535031473309));
#9483=CARTESIAN_POINT('Ctrl Pts',(86.8688358088513,4.39625599797244,-0.87971736114577));
#9484=CARTESIAN_POINT('Ctrl Pts',(87.0363251158703,3.13369152781732,3.20639156119395));
#9485=CARTESIAN_POINT('Ctrl Pts',(87.2038144228895,-0.980294174077118,4.37492774425823));
#9486=CARTESIAN_POINT('Ctrl Pts',(87.3713037299086,-4.20228664801629,1.56261203218003));
#9487=CARTESIAN_POINT('Ctrl Pts',(87.5387930369276,-3.60051750928825,-2.67156192152051));
#9488=CARTESIAN_POINT('Ctrl Pts',(87.7062823439467,0.277449040735304,-4.47481747840133));
#9489=CARTESIAN_POINT('Ctrl Pts',(87.8737716509658,3.90295804078757,-2.20632907043807));
#9490=CARTESIAN_POINT('Ctrl Pts',(88.0412609579849,3.97707172151794,2.06975118241549));
#9491=CARTESIAN_POINT('Ctrl Pts',(88.2087502650039,0.432352263689362,4.46251509300548));
#9492=CARTESIAN_POINT('Ctrl Pts',(88.376239572023,-3.50577490939459,2.79472927487746));
#9493=CARTESIAN_POINT('Ctrl Pts',(88.5437288790421,-4.25391323973235,-1.41604787490757));
#9494=CARTESIAN_POINT('Ctrl Pts',(88.7112181860611,-1.13131368088138,-4.33832903209606));
#9495=CARTESIAN_POINT('Ctrl Pts',(88.8787074930802,3.0206953845475,-3.31306034187067));
#9496=CARTESIAN_POINT('Ctrl Pts',(89.0461968000993,4.42410112458583,0.726841574634959));
#9497=CARTESIAN_POINT('Ctrl Pts',(89.2136861071185,1.80191092895468,4.10537287463695));
#9498=CARTESIAN_POINT('Ctrl Pts',(89.3811754141374,-2.45988132542442,3.74832673324009));
#9499=CARTESIAN_POINT('Ctrl Pts',(89.5486647211567,-4.48336844461608,-0.019411984135895));
#9500=CARTESIAN_POINT('Ctrl Pts',(89.7161540281755,-2.42733086926145,-3.76948727145864));
#9501=CARTESIAN_POINT('Ctrl Pts',(89.8836433351947,1.83739339888565,-4.08961549847513));
#9502=CARTESIAN_POINT('Ctrl Pts',(90.0511326422138,4.43022925631431,-0.68850430279645));
#9503=CARTESIAN_POINT('Ctrl Pts',(90.2186219492329,2.99189304342021,3.33909351087369));
#9504=CARTESIAN_POINT('Ctrl Pts',(90.3861112562519,-1.16883855184235,4.32836987953842));
#9505=CARTESIAN_POINT('Ctrl Pts',(90.5536005632711,-4.26601585988102,1.37915849781332));
#9506=CARTESIAN_POINT('Ctrl Pts',(90.72108987029,-3.48144281131612,-2.82498239452599));
#9507=CARTESIAN_POINT('Ctrl Pts',(90.8885791773093,0.470978714292056,-4.45860381844503));
#9508=CARTESIAN_POINT('Ctrl Pts',(91.0560684843282,3.99484539860717,-2.03523466585599));
#9509=CARTESIAN_POINT('Ctrl Pts',(91.2235577913474,3.88370622939613,2.24004379457078));
#9510=CARTESIAN_POINT('Ctrl Pts',(91.3910470983663,0.238689464243757,4.47705183611538));
#9511=CARTESIAN_POINT('Ctrl Pts',(91.5585364053856,-3.62351665470846,2.64028426831555));
#9512=CARTESIAN_POINT('Ctrl Pts',(91.7260257124045,-4.18859774141264,-1.59894426869731));
#9513=CARTESIAN_POINT('Ctrl Pts',(91.8935150194237,-0.942373367957906,-4.38324934993722));
#9514=CARTESIAN_POINT('Ctrl Pts',(92.0610043264428,3.16133974716656,-3.17914162246129));
#9515=CARTESIAN_POINT('Ctrl Pts',(92.2284936334618,4.3884727345685,0.917765380581216));
#9516=CARTESIAN_POINT('Ctrl Pts',(92.3959829404809,1.62243111591272,4.17953241833476));
#9517=CARTESIAN_POINT('Ctrl Pts',(92.5634722475,-2.61990390537629,3.63832759739651));
#9518=CARTESIAN_POINT('Ctrl Pts',(92.7309615545189,-4.47831684710423,-0.213646755827483));
#9519=CARTESIAN_POINT('Ctrl Pts',(92.8984508615383,-2.26181852338362,-3.8708880009044));
#9520=CARTESIAN_POINT('Ctrl Pts',(93.0659401685571,2.012796057528,-4.00656729179735));
#9521=CARTESIAN_POINT('Ctrl Pts',(93.2334294755763,4.45585371659675,-0.495289157095007));
#9522=CARTESIAN_POINT('Ctrl Pts',(93.4009187825954,2.84455105545746,3.46412782770724));
#9523=CARTESIAN_POINT('Ctrl Pts',(93.5684080896144,-1.35531917368203,4.27648182274434));
#9524=CARTESIAN_POINT('Ctrl Pts',(93.7358973966335,-4.32158983383552,1.18730386515585));
#9525=CARTESIAN_POINT('Ctrl Pts',(93.8475569346462,-3.67692205783178,-1.57603342148763));
#9526=CARTESIAN_POINT('Ctrl Pts',(93.9033867036526,-2.84228154559889,-2.5181189220424));
#9527=CARTESIAN_POINT('Ctrl Pts',(75.0455976138633,3.06645132020445,-2.51949456504998));
#9528=CARTESIAN_POINT('Ctrl Pts',(75.1014273828696,3.90154779477274,-1.50310710287372));
#9529=CARTESIAN_POINT('Ctrl Pts',(75.2130869208824,4.46742805898946,1.40805985264505));
#9530=CARTESIAN_POINT('Ctrl Pts',(75.3805762279014,1.24927847597423,4.51916377824188));
#9531=CARTESIAN_POINT('Ctrl Pts',(75.5480655349206,-3.10559897573176,3.50744378058995));
#9532=CARTESIAN_POINT('Ctrl Pts',(75.7155548419395,-4.63455987727541,-0.69052054092898));
#9533=CARTESIAN_POINT('Ctrl Pts',(75.8830441489587,-1.9464585018686,-4.26281795947025));
#9534=CARTESIAN_POINT('Ctrl Pts',(76.0505334559777,2.51279058774102,-3.9549296545997));
#9535=CARTESIAN_POINT('Ctrl Pts',(76.2180227629969,4.68558178106048,-0.0490381362345196));
#9536=CARTESIAN_POINT('Ctrl Pts',(76.3855120700159,2.59485425351327,3.90182050286693));
#9537=CARTESIAN_POINT('Ctrl Pts',(76.553001377035,-1.85699592939576,4.30214329460675));
#9538=CARTESIAN_POINT('Ctrl Pts',(76.720490684054,-4.61911966559588,0.787931595618742));
#9539=CARTESIAN_POINT('Ctrl Pts',(76.8879799910731,-3.17819602892282,-3.44328319184127));
#9540=CARTESIAN_POINT('Ctrl Pts',(77.0554692980923,1.15464486915952,-4.54134892492803));
#9541=CARTESIAN_POINT('Ctrl Pts',(77.2229586051112,4.43684649216151,-1.50714376233198));
#9542=CARTESIAN_POINT('Ctrl Pts',(77.3904479121304,3.68185494419516,2.8984536307935));
#9543=CARTESIAN_POINT('Ctrl Pts',(77.5579372191495,-0.423344942904035,4.66667541455828));
#9544=CARTESIAN_POINT('Ctrl Pts',(77.7254265261685,-4.14333307156369,2.18857860516851));
#9545=CARTESIAN_POINT('Ctrl Pts',(77.8929158331877,-4.09320287414477,-2.28095924459537));
#9546=CARTESIAN_POINT('Ctrl Pts',(78.0604051402067,-0.318569006102588,-4.67499706960582));
#9547=CARTESIAN_POINT('Ctrl Pts',(78.2278944472258,3.74593845389551,-2.81514290719053));
#9548=CARTESIAN_POINT('Ctrl Pts',(78.3953837542449,4.40192649164485,1.60627754211177));
#9549=CARTESIAN_POINT('Ctrl Pts',(78.5628730612639,1.05249582445596,4.56610740188116));
#9550=CARTESIAN_POINT('Ctrl Pts',(78.7303623682829,-3.25462608720204,3.37112642739182));
#9551=CARTESIAN_POINT('Ctrl Pts',(78.8978516753021,-4.60028550535166,-0.891323513257688));
#9552=CARTESIAN_POINT('Ctrl Pts',(79.065340982321,-1.76003458552832,-4.34273676176006));
#9553=CARTESIAN_POINT('Ctrl Pts',(79.2328302893404,2.68171410172883,-3.84258946710639));
#9554=CARTESIAN_POINT('Ctrl Pts',(79.4003195963591,4.6833066794353,0.154022332581167));
#9555=CARTESIAN_POINT('Ctrl Pts',(79.5678089033785,2.42344595773958,4.01048550943476));
#9556=CARTESIAN_POINT('Ctrl Pts',(79.7352982103974,-2.04156648246805,4.21771153952704));
#9557=CARTESIAN_POINT('Ctrl Pts',(79.9027875174165,-4.64890851624551,0.58714047724318));
#9558=CARTESIAN_POINT('Ctrl Pts',(80.0702768244356,-3.0260969659929,-3.57768381564977));
#9559=CARTESIAN_POINT('Ctrl Pts',(80.2377661314547,1.35023293842321,-4.48708762389827));
#9560=CARTESIAN_POINT('Ctrl Pts',(80.4052554384738,4.49795344263644,-1.3135825670034));
#9561=CARTESIAN_POINT('Ctrl Pts',(80.5727447454928,3.55287801213224,3.05518283632336));
#9562=CARTESIAN_POINT('Ctrl Pts',(80.7402340525119,-0.625046506306802,4.64396395307223));
#9563=CARTESIAN_POINT('Ctrl Pts',(80.907723359531,-4.23422618719991,2.00709066265056));
#9564=CARTESIAN_POINT('Ctrl Pts',(81.07521266655,-3.99058170113424,-2.45608265720882));
#9565=CARTESIAN_POINT('Ctrl Pts',(81.2427019735693,-0.115811021377698,-4.68440734136128));
#9566=CARTESIAN_POINT('Ctrl Pts',(81.4101912805881,3.86433888996382,-2.65027720738482));
#9567=CARTESIAN_POINT('Ctrl Pts',(81.5776805876074,4.32823397543431,1.79540385049343));
#9568=CARTESIAN_POINT('Ctrl Pts',(81.7451698946263,0.853764948185291,4.60740379668648));
#9569=CARTESIAN_POINT('Ctrl Pts',(81.9126592016455,-3.39756532356089,3.2270163006417));
#9570=CARTESIAN_POINT('Ctrl Pts',(82.0801485086645,-4.55736925526216,-1.08971088076697));
#9571=CARTESIAN_POINT('Ctrl Pts',(82.2476378156836,-1.57031337642494,-4.4148839432415));
#9572=CARTESIAN_POINT('Ctrl Pts',(82.4151271227027,2.84560838224604,-3.72284800486962));
#9573=CARTESIAN_POINT('Ctrl Pts',(82.5826164297219,4.67224268670378,0.3566968026402));
#9574=CARTESIAN_POINT('Ctrl Pts',(82.7501057367407,2.24749108465355,4.11167461709625));
#9575=CARTESIAN_POINT('Ctrl Pts',(82.9175950437602,-2.22230666825049,4.1253408834568));
#9576=CARTESIAN_POINT('Ctrl Pts',(83.0850843507788,-4.66997417603144,0.385260337525263));
#9577=CARTESIAN_POINT('Ctrl Pts',(83.2525736577983,-2.86831994968329,-3.70537784830637));
#9578=CARTESIAN_POINT('Ctrl Pts',(83.4200629648169,1.54328753190602,-4.42440368030926));
#9579=CARTESIAN_POINT('Ctrl Pts',(83.5875522718364,4.5506205990891,-1.11755827392429));
#9580=CARTESIAN_POINT('Ctrl Pts',(83.7550415788553,3.41723462017294,3.20618026367237));
#9581=CARTESIAN_POINT('Ctrl Pts',(83.9225308858744,-0.825575264478656,4.61253832668647));
#9582=CARTESIAN_POINT('Ctrl Pts',(84.0900201928935,-4.31717437530757,1.82183691522002));
#9583=CARTESIAN_POINT('Ctrl Pts',(84.2575094999126,-3.88047276936262,-2.62659768878029));
#9584=CARTESIAN_POINT('Ctrl Pts',(84.4249988069316,0.0871642670565068,-4.68502793193585));
#9585=CARTESIAN_POINT('Ctrl Pts',(84.5924881139508,3.97548844210186,-2.48043866668484));
#9586=CARTESIAN_POINT('Ctrl Pts',(84.7599774209698,4.24642014257932,1.9811613526332));
#9587=CARTESIAN_POINT('Ctrl Pts',(84.9274667279889,0.653432103046516,4.64005504484363));
#9588=CARTESIAN_POINT('Ctrl Pts',(85.0949560350079,-3.53412951068382,3.07685113942557));
#9589=CARTESIAN_POINT('Ctrl Pts',(85.262445342027,-4.50590174852132,-1.28605356231507));
#9590=CARTESIAN_POINT('Ctrl Pts',(85.4299346490461,-1.37764569709891,-4.47874722056687));
#9591=CARTESIAN_POINT('Ctrl Pts',(85.5974239560652,3.0041632824441,-3.59612114713693));
#9592=CARTESIAN_POINT('Ctrl Pts',(85.7649132630843,4.65241189360609,0.558701982011273));
#9593=CARTESIAN_POINT('Ctrl Pts',(85.9324025701033,2.06731911348409,4.20514875069765));
#9594=CARTESIAN_POINT('Ctrl Pts',(86.0998918771224,-2.39887701093383,4.02522961070344));
#9595=CARTESIAN_POINT('Ctrl Pts',(86.2673811841415,-4.68227729198668,0.182657311423967));
#9596=CARTESIAN_POINT('Ctrl Pts',(86.4348704911605,-2.70516093802755,-3.82611926523999));
#9597=CARTESIAN_POINT('Ctrl Pts',(86.6023597981797,1.7334463653411,-4.35341797108391));
#9598=CARTESIAN_POINT('Ctrl Pts',(86.7698491051987,4.59474916176048,-0.919437041331279));
#9599=CARTESIAN_POINT('Ctrl Pts',(86.9373384122179,3.27517927238433,3.35116174873949));
#9600=CARTESIAN_POINT('Ctrl Pts',(87.1048277192368,-1.02455494782308,4.5724579266913));
#9601=CARTESIAN_POINT('Ctrl Pts',(87.2723170262561,-4.39202199834478,1.63316474935204));
#9602=CARTESIAN_POINT('Ctrl Pts',(87.439806333275,-3.7630826811123,-2.79218428252561));
#9603=CARTESIAN_POINT('Ctrl Pts',(87.6072956402942,0.289976004112983,-4.67685773244287));
#9604=CARTESIAN_POINT('Ctrl Pts',(87.7747849473131,4.07917855433484,-2.3059459348224));
#9605=CARTESIAN_POINT('Ctrl Pts',(87.9422742543323,4.15663850493095,2.16320148663827));
#9606=CARTESIAN_POINT('Ctrl Pts',(88.1097635613514,0.451873185294068,4.66399988817462));
#9607=CARTESIAN_POINT('Ctrl Pts',(88.2772528683704,-3.66406240530372,2.92091270367628));
#9608=CARTESIAN_POINT('Ctrl Pts',(88.4447421753896,-4.44597955657645,-1.47998314685156));
#9609=CARTESIAN_POINT('Ctrl Pts',(88.6122314824085,-1.18239306112185,-4.53420676431444));
#9610=CARTESIAN_POINT('Ctrl Pts',(88.7797207894278,3.15708129655885,-3.46264667837653));
#9611=CARTESIAN_POINT('Ctrl Pts',(88.9472100964467,4.6238515098096,0.75965883636597));
#9612=CARTESIAN_POINT('Ctrl Pts',(89.1146994034659,1.88326811136568,4.29073251947842));
#9613=CARTESIAN_POINT('Ctrl Pts',(89.2821887104849,-2.57094620132151,3.91756556567735));
#9614=CARTESIAN_POINT('Ctrl Pts',(89.4496780175041,-4.68579477907199,-0.0202884449580863));
#9615=CARTESIAN_POINT('Ctrl Pts',(89.617167324523,-2.53692607573313,-3.93968151281212));
#9616=CARTESIAN_POINT('Ctrl Pts',(89.7846566315422,1.9203526326146,-4.27426368987786));
#9617=CARTESIAN_POINT('Ctrl Pts',(89.9521459385612,4.63025632975995,-0.719590617471205));
#9618=CARTESIAN_POINT('Ctrl Pts',(90.1196352455803,3.12697851528032,3.48985525802016));
#9619=CARTESIAN_POINT('Ctrl Pts',(90.2871245525994,-1.22161219883188,4.5237979510226));
#9620=CARTESIAN_POINT('Ctrl Pts',(90.4546138596185,-4.45862861609638,1.44142819587512));
#9621=CARTESIAN_POINT('Ctrl Pts',(90.6221031666375,-3.63863170079026,-2.95253176685409));
#9622=CARTESIAN_POINT('Ctrl Pts',(90.7895924736566,0.492243639519289,-4.6599120176056));
#9623=CARTESIAN_POINT('Ctrl Pts',(90.9570817806758,4.17521467245732,-2.12712653204012));
#9624=CARTESIAN_POINT('Ctrl Pts',(91.1245710876947,4.05905751400097,2.34118289566344));
#9625=CARTESIAN_POINT('Ctrl Pts',(91.2920603947138,0.249466413298239,4.67919297252862));
#9626=CARTESIAN_POINT('Ctrl Pts',(91.4595497017329,-3.78712024948626,2.75949442758732));
#9627=CARTESIAN_POINT('Ctrl Pts',(91.6270390087521,-4.37771503074064,-1.67113740457495));
#9628=CARTESIAN_POINT('Ctrl Pts',(91.7945283157709,-0.984921998283766,-4.58115525704141));
#9629=CARTESIAN_POINT('Ctrl Pts',(91.9620176227903,3.30407582270753,-3.32268146160252));
#9630=CARTESIAN_POINT('Ctrl Pts',(92.1295069298092,4.58661448010922,0.959202947931876));
#9631=CARTESIAN_POINT('Ctrl Pts',(92.2969962368283,1.69568469472483,4.36824040377796));
#9632=CARTESIAN_POINT('Ctrl Pts',(92.4644855438475,-2.73819388103709,3.80259991366693));
#9633=CARTESIAN_POINT('Ctrl Pts',(92.6319748508664,-4.68051509939824,-0.22329301403374));
#9634=CARTESIAN_POINT('Ctrl Pts',(92.7994641578856,-2.36394076440595,-4.0456605360623));
#9635=CARTESIAN_POINT('Ctrl Pts',(92.9669534649047,2.10367480928929,-4.18746581500559));
#9636=CARTESIAN_POINT('Ctrl Pts',(93.1344427719237,4.65703774727922,-0.51765171101067));
#9637=CARTESIAN_POINT('Ctrl Pts',(93.3019320789428,2.97298396264366,3.62053493698499));
#9638=CARTESIAN_POINT('Ctrl Pts',(93.4694213859619,-1.41651251429978,4.46956712243346));
#9639=CARTESIAN_POINT('Ctrl Pts',(93.6369106929809,-4.51671178285486,1.24091123030503));
#9640=CARTESIAN_POINT('Ctrl Pts',(93.7485702309937,-3.84293693335262,-1.64719212112001));
#9641=CARTESIAN_POINT('Ctrl Pts',(93.8044,-2.97061198327643,-2.63181325464298));
#9642=CARTESIAN_POINT('Ctrl Pts',(75.342557724821,2.66903922910601,-2.19296806941944));
#9643=CARTESIAN_POINT('Ctrl Pts',(75.342557724821,2.74445357713776,-2.11551288776751));
#9644=CARTESIAN_POINT('Ctrl Pts',(75.342557724821,2.81573387113398,-2.03445442488076));
#9645=CARTESIAN_POINT('Ctrl Pts',(75.342557724821,2.88288676332201,-1.95020526406688));
#9646=CARTESIAN_POINT('Ctrl Pts',(75.342557724821,2.95167275371243,-1.8639072391074));
#9647=CARTESIAN_POINT('Ctrl Pts',(75.342557724821,3.01612853799601,-1.77426095588347));
#9648=CARTESIAN_POINT('Ctrl Pts',(75.342557724821,3.07622945879123,-1.68166519380833));
#9649=CARTESIAN_POINT('Ctrl Pts',(75.342557724821,3.13744571756752,-1.58735106254747));
#9650=CARTESIAN_POINT('Ctrl Pts',(75.342557724821,3.19414439702615,-1.48997634213879));
#9651=CARTESIAN_POINT('Ctrl Pts',(75.342557724821,3.24626072027771,-1.38992521171123));
#9652=CARTESIAN_POINT('Ctrl Pts',(75.342557724821,3.25521273849457,-1.37273943408296));
#9653=CARTESIAN_POINT('Ctrl Pts',(75.342557724821,3.2640294549757,-1.35547461535056));
#9654=CARTESIAN_POINT('Ctrl Pts',(75.342557724821,3.27271041500071,-1.33813261632123));
#9655=CARTESIAN_POINT('Ctrl Pts',(75.342557724821,3.28114951999669,-1.32127377234235));
#9656=CARTESIAN_POINT('Ctrl Pts',(75.342557724821,3.28945668002034,-1.30434921737686));
#9657=CARTESIAN_POINT('Ctrl Pts',(75.342557724821,3.29762966865746,-1.28736537979867));
#9658=CARTESIAN_POINT('Ctrl Pts',(75.342557724821,3.34731909381879,-1.18410852190207));
#9659=CARTESIAN_POINT('Ctrl Pts',(75.342557724821,3.39207834736118,-1.07861149239416));
#9660=CARTESIAN_POINT('Ctrl Pts',(75.342557724821,3.43188270629604,-0.971303217913125));
#9661=CARTESIAN_POINT('Ctrl Pts',(75.342557724821,3.47217664595643,-0.862675086404327));
#9662=CARTESIAN_POINT('Ctrl Pts',(75.342557724821,3.50739344417012,-0.752190133416963));
#9663=CARTESIAN_POINT('Ctrl Pts',(75.342557724821,3.53746516435151,-0.640259734304225));
#9664=CARTESIAN_POINT('Ctrl Pts',(75.342557724821,3.5568869054314,-0.567969781570485));
#9665=CARTESIAN_POINT('Ctrl Pts',(75.342557724821,3.57416166527878,-0.495076252130135));
#9666=CARTESIAN_POINT('Ctrl Pts',(75.342557724821,3.58926077368719,-0.421684949048237));
#9667=CARTESIAN_POINT('Ctrl Pts',(75.342557724821,3.59566205252182,-0.390570648630151));
#9668=CARTESIAN_POINT('Ctrl Pts',(75.342557724821,3.60167218796151,-0.359366843973714));
#9669=CARTESIAN_POINT('Ctrl Pts',(75.342557724821,3.60728852407918,-0.32808146002479));
#9670=CARTESIAN_POINT('Ctrl Pts',(75.342557724821,3.61050399245623,-0.310169931824944));
#9671=CARTESIAN_POINT('Ctrl Pts',(75.342557724821,3.61359044725664,-0.292230814311455));
#9672=CARTESIAN_POINT('Ctrl Pts',(75.342557724821,3.61654486489718,-0.274281913907966));
#9673=CARTESIAN_POINT('Ctrl Pts',(75.342557724821,3.63581733262553,-0.157196367491248));
#9674=CARTESIAN_POINT('Ctrl Pts',(75.342557724821,3.64950486260566,-0.0395354677081342));
#9675=CARTESIAN_POINT('Ctrl Pts',(75.342557724821,3.65756797097238,0.0782629527285851));
#9676=CARTESIAN_POINT('Ctrl Pts',(75.342557724821,3.66562084842487,0.195911904067305));
#9677=CARTESIAN_POINT('Ctrl Pts',(75.342557724821,3.66806386102843,0.313698907639059));
#9678=CARTESIAN_POINT('Ctrl Pts',(75.342557724821,3.66481050835095,0.431210226129204));
#9679=CARTESIAN_POINT('Ctrl Pts',(75.342557724821,3.66155095575816,0.548945485979381));
#9680=CARTESIAN_POINT('Ctrl Pts',(75.342557724821,3.652573642136,0.666404895833316));
#9681=CARTESIAN_POINT('Ctrl Pts',(75.342557724821,3.6377394439107,0.783181642415076));
#9682=CARTESIAN_POINT('Ctrl Pts',(75.342557724821,3.63032234479805,0.841570015705956));
#9683=CARTESIAN_POINT('Ctrl Pts',(75.342557724821,3.62144017952809,0.899787785327359));
#9684=CARTESIAN_POINT('Ctrl Pts',(75.342557724821,3.61107027366315,0.957783896510187));
#9685=CARTESIAN_POINT('Ctrl Pts',(75.342557724821,3.60549862512678,0.988944637233916));
#9686=CARTESIAN_POINT('Ctrl Pts',(75.342557724821,3.59949743250429,1.02004138237487));
#9687=CARTESIAN_POINT('Ctrl Pts',(75.342557724821,3.59306273653391,1.05106613735378));
#9688=CARTESIAN_POINT('Ctrl Pts',(75.342557724821,3.58935704516694,1.06893305246783));
#9689=CARTESIAN_POINT('Ctrl Pts',(75.342557724821,3.5855075758258,1.08677609073766));
#9690=CARTESIAN_POINT('Ctrl Pts',(75.342557724821,3.58151352449986,1.10459371393155));
#9691=CARTESIAN_POINT('Ctrl Pts',(75.342557724821,3.57953485452689,1.11342064005904));
#9692=CARTESIAN_POINT('Ctrl Pts',(75.342557724821,3.57752094215402,1.12224021146939));
#9693=CARTESIAN_POINT('Ctrl Pts',(75.342557724821,3.57547241467767,1.13104933483286));
#9694=CARTESIAN_POINT('Ctrl Pts',(75.342557724821,3.54994667569026,1.24081568470107));
#9695=CARTESIAN_POINT('Ctrl Pts',(75.342557724821,3.51902110526928,1.34909263168916));
#9696=CARTESIAN_POINT('Ctrl Pts',(75.342557724821,3.4830615869259,1.45565358445287));
#9697=CARTESIAN_POINT('Ctrl Pts',(75.342557724821,3.4456917452281,1.56639383124708));
#9698=CARTESIAN_POINT('Ctrl Pts',(75.342557724821,3.40288528203317,1.67528140979421));
#9699=CARTESIAN_POINT('Ctrl Pts',(75.342557724821,3.35499628463391,1.78206193622134));
#9700=CARTESIAN_POINT('Ctrl Pts',(75.342557724821,3.30622973510779,1.89079918513508));
#9701=CARTESIAN_POINT('Ctrl Pts',(75.342557724821,3.25219236001142,1.99735212957777));
#9702=CARTESIAN_POINT('Ctrl Pts',(75.342557724821,3.19320376567024,2.10144246943319));
#9703=CARTESIAN_POINT('Ctrl Pts',(75.342557724821,3.15375302502262,2.17105662192186));
#9704=CARTESIAN_POINT('Ctrl Pts',(75.342557724821,3.11208660904809,2.23956910381198));
#9705=CARTESIAN_POINT('Ctrl Pts',(75.342557724821,3.06828808096117,2.30689197306326));
#9706=CARTESIAN_POINT('Ctrl Pts',(75.342557724821,3.04770324685026,2.33853299288607));
#9707=CARTESIAN_POINT('Ctrl Pts',(75.342557724821,3.02664732063322,2.36991117398798));
#9708=CARTESIAN_POINT('Ctrl Pts',(75.342557724821,3.00512831524903,2.40101699498357));
#9709=CARTESIAN_POINT('Ctrl Pts',(75.342557724821,2.99490091546237,2.41580074829069));
#9710=CARTESIAN_POINT('Ctrl Pts',(75.342557724821,2.98456791657202,2.43052436587747));
#9711=CARTESIAN_POINT('Ctrl Pts',(75.342557724821,2.9741332515261,2.4451824474385));
#9712=CARTESIAN_POINT('Ctrl Pts',(75.342557724821,2.90048108769345,2.54864522461958));
#9713=CARTESIAN_POINT('Ctrl Pts',(75.3425577248209,2.82202212090033,2.64849018376099));
#9714=CARTESIAN_POINT('Ctrl Pts',(75.3425577248209,2.7391739809035,2.74441746113153));
#9715=CARTESIAN_POINT('Ctrl Pts',(75.3425577248209,2.65815137026194,2.83823101499762));
#9716=CARTESIAN_POINT('Ctrl Pts',(75.3425577248209,2.57293010747928,2.92829830822171));
#9717=CARTESIAN_POINT('Ctrl Pts',(75.3425577248209,2.48384819044702,3.01432170978502));
#9718=CARTESIAN_POINT('Ctrl Pts',(75.3425577248209,2.39175560170328,3.10325241543698));
#9719=CARTESIAN_POINT('Ctrl Pts',(75.3425577248209,2.29553663680206,3.18786226001191));
#9720=CARTESIAN_POINT('Ctrl Pts',(75.3425577248209,2.19551580562984,3.26779099829018));
#9721=CARTESIAN_POINT('Ctrl Pts',(75.3425577248209,2.09549497445763,3.34771973656845));
#9722=CARTESIAN_POINT('Ctrl Pts',(75.3425577248209,1.99167161659826,3.42296825978045));
#9723=CARTESIAN_POINT('Ctrl Pts',(75.3425577248209,1.88433026752066,3.49313140215102));
#9724=CARTESIAN_POINT('Ctrl Pts',(77.0459088298365,-3.45658164681457,0.00280094662916092));
#9725=CARTESIAN_POINT('Ctrl Pts',(77.0364228182283,-3.45828790519784,0.196977771036481));
#9726=CARTESIAN_POINT('Ctrl Pts',(77.02693680662,-3.44332490726161,0.390891484629403));
#9727=CARTESIAN_POINT('Ctrl Pts',(77.0174507950117,-3.41075968470985,0.581802412792217));
#9728=CARTESIAN_POINT('Ctrl Pts',(76.9616210260054,-3.21909759027179,1.70540561509294));
#9729=CARTESIAN_POINT('Ctrl Pts',(76.905791256999,-2.41771342360892,2.72499556935934));
#9730=CARTESIAN_POINT('Ctrl Pts',(76.8499614879927,-1.37120627374349,3.17671705350414));
#9731=CARTESIAN_POINT('Ctrl Pts',(76.7941317189863,-0.324699123878052,3.62843853764894));
#9732=CARTESIAN_POINT('Ctrl Pts',(76.7383019499799,0.966931009189941,3.51229155167215));
#9733=CARTESIAN_POINT('Ctrl Pts',(76.6824721809736,1.91604094905346,2.88108016543812));
#9734=CARTESIAN_POINT('Ctrl Pts',(76.6266424119672,2.86515088891698,2.24986877920407));
#9735=CARTESIAN_POINT('Ctrl Pts',(76.5708126429609,3.47174063557601,1.10359299271277));
#9736=CARTESIAN_POINT('Ctrl Pts',(76.5149828739545,3.45983593312798,-0.0361595634637213));
#9737=CARTESIAN_POINT('Ctrl Pts',(76.4591531049482,3.44793123067995,-1.17591211964021));
#9738=CARTESIAN_POINT('Ctrl Pts',(76.4033233359418,2.81753207912487,-2.3091414455019));
#9739=CARTESIAN_POINT('Ctrl Pts',(76.3474935669354,1.85544410208129,-2.92042043852596));
#9740=CARTESIAN_POINT('Ctrl Pts',(76.291663797929,0.89335612503771,-3.53169943155002));
#9741=CARTESIAN_POINT('Ctrl Pts',(76.2358340289227,-0.400420677494361,-3.62102809173647));
#9742=CARTESIAN_POINT('Ctrl Pts',(76.1800042599164,-1.43726298495274,-3.14747114297997));
#9743=CARTESIAN_POINT('Ctrl Pts',(76.12417449091,-2.47410529241112,-2.67391419422347));
#9744=CARTESIAN_POINT('Ctrl Pts',(76.0683447219036,-3.25401310479582,-1.63747163652403));
#9745=CARTESIAN_POINT('Ctrl Pts',(76.0125149528973,-3.42216574953757,-0.510265666765961));
#9746=CARTESIAN_POINT('Ctrl Pts',(76.0042018007659,-3.44720397810103,-0.34242268842772));
#9747=CARTESIAN_POINT('Ctrl Pts',(75.9958886486346,-3.4586785296033,-0.172567327235602));
#9748=CARTESIAN_POINT('Ctrl Pts',(75.9875754965032,-3.45725565822888,-0.00252520199929829));
#9749=CARTESIAN_POINT('Origin',(75.342557724821,-5.12956166756098E-16,0.));
#9750=CARTESIAN_POINT('Ctrl Pts',(75.342557724821,-1.88729338390967,3.49128919534759));
#9751=CARTESIAN_POINT('Ctrl Pts',(75.342557724821,-1.98965881273553,3.42582705186126));
#9752=CARTESIAN_POINT('Ctrl Pts',(75.342557724821,-2.08853316026797,3.3554367053497));
#9753=CARTESIAN_POINT('Ctrl Pts',(75.342557724821,-2.18376353031218,3.28051395785925));
#9754=CARTESIAN_POINT('Ctrl Pts',(75.342557724821,-2.28075909933827,3.20420243536427));
#9755=CARTESIAN_POINT('Ctrl Pts',(75.342557724821,-2.37397483745187,3.12318822942394));
#9756=CARTESIAN_POINT('Ctrl Pts',(75.342557724821,-2.46321093678954,3.03785174096976));
#9757=CARTESIAN_POINT('Ctrl Pts',(75.342557724821,-2.55600352323115,2.94911418363274));
#9758=CARTESIAN_POINT('Ctrl Pts',(75.342557724821,-2.64449370202301,2.85570220672163));
#9759=CARTESIAN_POINT('Ctrl Pts',(75.342557724821,-2.72840589024478,2.75801402183562));
#9760=CARTESIAN_POINT('Ctrl Pts',(75.342557724821,-2.74149425994018,2.74277691378545));
#9761=CARTESIAN_POINT('Ctrl Pts',(75.342557724821,-2.75447114178973,2.72743572798769));
#9762=CARTESIAN_POINT('Ctrl Pts',(75.342557724821,-2.76733536476255,2.71199193333328));
#9763=CARTESIAN_POINT('Ctrl Pts',(75.342557724821,-2.78020766002005,2.69653844771603));
#9764=CARTESIAN_POINT('Ctrl Pts',(75.342557724821,-2.79296228879439,2.68098801714063));
#9765=CARTESIAN_POINT('Ctrl Pts',(75.342557724821,-2.80559444421283,2.66534725776366));
#9766=CARTESIAN_POINT('Ctrl Pts',(75.342557724821,-2.88250675556822,2.57011671988728));
#9767=CARTESIAN_POINT('Ctrl Pts',(75.342557724821,-2.95492997736749,2.47148290468358));
#9768=CARTESIAN_POINT('Ctrl Pts',(75.342557724821,-3.02267228602371,2.36982066191873));
#9769=CARTESIAN_POINT('Ctrl Pts',(75.342557724821,-3.09007944726784,2.26866138160448));
#9770=CARTESIAN_POINT('Ctrl Pts',(75.342557724821,-3.15285221813227,2.16450273906243));
#9771=CARTESIAN_POINT('Ctrl Pts',(75.342557724821,-3.21075473121433,2.05769343219054));
#9772=CARTESIAN_POINT('Ctrl Pts',(75.342557724821,-3.24743521561524,1.99003113385415));
#9773=CARTESIAN_POINT('Ctrl Pts',(75.342557724821,-3.28216028458533,1.92130473789008));
#9774=CARTESIAN_POINT('Ctrl Pts',(75.342557724821,-3.3148592707336,1.85160082777986));
#9775=CARTESIAN_POINT('Ctrl Pts',(75.342557724821,-3.33199284148589,1.81507746677503));
#9776=CARTESIAN_POINT('Ctrl Pts',(75.342557724821,-3.34857000106658,1.77828570999916));
#9777=CARTESIAN_POINT('Ctrl Pts',(75.342557724821,-3.36457961037642,1.74123797347753));
#9778=CARTESIAN_POINT('Ctrl Pts',(75.342557724821,-3.37260637694873,1.7226632832814));
#9779=CARTESIAN_POINT('Ctrl Pts',(75.342557724821,-3.38049087856411,1.70402302661623));
#9780=CARTESIAN_POINT('Ctrl Pts',(75.342557724821,-3.38822413051831,1.68533759572285));
#9781=CARTESIAN_POINT('Ctrl Pts',(75.342557724821,-3.43394894182751,1.57485525182781));
#9782=CARTESIAN_POINT('Ctrl Pts',(75.342557724821,-3.47445615533811,1.46264468374345));
#9783=CARTESIAN_POINT('Ctrl Pts',(75.342557724821,-3.50955062331665,1.3490487877896));
#9784=CARTESIAN_POINT('Ctrl Pts',(75.342557724821,-3.54398194376743,1.23759940785103));
#9785=CARTESIAN_POINT('Ctrl Pts',(75.342557724821,-3.57320329370337,1.12481579109674));
#9786=CARTESIAN_POINT('Ctrl Pts',(75.342557724821,-3.59698123988467,1.01101268319051));
#9787=CARTESIAN_POINT('Ctrl Pts',(75.342557724821,-3.62144613123762,0.893921802030013));
#9788=CARTESIAN_POINT('Ctrl Pts',(75.342557724821,-3.64014916389457,0.77575088847576));
#9789=CARTESIAN_POINT('Ctrl Pts',(75.342557724821,-3.65277727238172,0.656844752533057));
#9790=CARTESIAN_POINT('Ctrl Pts',(75.342557724821,-3.65909132662529,0.597391684561706));
#9791=CARTESIAN_POINT('Ctrl Pts',(75.342557724821,-3.66388568603325,0.537754916717839));
#9792=CARTESIAN_POINT('Ctrl Pts',(75.342557724821,-3.66711521089121,0.477978690984206));
#9793=CARTESIAN_POINT('Ctrl Pts',(75.342557724821,-3.6688033537149,0.446732358803051));
#9794=CARTESIAN_POINT('Ctrl Pts',(75.342557724821,-3.67006385615744,0.415447938173428));
#9795=CARTESIAN_POINT('Ctrl Pts',(75.342557724821,-3.67088981459646,0.384131877900408));
#9796=CARTESIAN_POINT('Ctrl Pts',(75.342557724821,-3.67138709308039,0.365277656865117));
#9797=CARTESIAN_POINT('Ctrl Pts',(75.342557724821,-3.67172685235443,0.346411968980907));
#9798=CARTESIAN_POINT('Ctrl Pts',(75.342557724821,-3.67190752969518,0.327536240136365));
#9799=CARTESIAN_POINT('Ctrl Pts',(75.342557724821,-3.6720008604043,0.317785791348867));
#9800=CARTESIAN_POINT('Ctrl Pts',(75.342557724821,-3.6720517296715,0.308032276855914));
#9801=CARTESIAN_POINT('Ctrl Pts',(75.342557724821,-3.67205995067616,0.298281359438954));
#9802=CARTESIAN_POINT('Ctrl Pts',(75.342557724821,-3.67215633969913,0.183954529334913));
#9803=CARTESIAN_POINT('Ctrl Pts',(75.342557724821,-3.66639691553994,0.0698132970449268));
#9804=CARTESIAN_POINT('Ctrl Pts',(75.342557724821,-3.65504660301135,-0.0437875909146339));
#9805=CARTESIAN_POINT('Ctrl Pts',(75.342557724821,-3.64352708680288,-0.15908197306051));
#9806=CARTESIAN_POINT('Ctrl Pts',(75.342557724821,-3.62624835841427,-0.273820618695414));
#9807=CARTESIAN_POINT('Ctrl Pts',(75.342557724821,-3.60343270120605,-0.38762384282797));
#9808=CARTESIAN_POINT('Ctrl Pts',(75.342557724821,-3.5805479808187,-0.501771550241523));
#9809=CARTESIAN_POINT('Ctrl Pts',(75.342557724821,-3.55209226834181,-0.614979001429506));
#9810=CARTESIAN_POINT('Ctrl Pts',(75.342557724821,-3.5182421068499,-0.726841589629112));
#9811=CARTESIAN_POINT('Ctrl Pts',(75.342557724821,-3.49759611478955,-0.795069155053657));
#9812=CARTESIAN_POINT('Ctrl Pts',(75.342557724821,-3.47494245755732,-0.862795951760317));
#9813=CARTESIAN_POINT('Ctrl Pts',(75.342557724821,-3.45031368885424,-0.92992425346773));
#9814=CARTESIAN_POINT('Ctrl Pts',(75.342557724821,-3.43733424954629,-0.965301081613749));
#9815=CARTESIAN_POINT('Ctrl Pts',(75.342557724821,-3.42380616879117,-1.00051160361389));
#9816=CARTESIAN_POINT('Ctrl Pts',(75.342557724821,-3.40973365029785,-1.03554089181167));
#9817=CARTESIAN_POINT('Ctrl Pts',(75.342557724821,-3.40339158387213,-1.05132755236583));
#9818=CARTESIAN_POINT('Ctrl Pts',(75.342557724821,-3.39693849996648,-1.06707827537105));
#9819=CARTESIAN_POINT('Ctrl Pts',(75.342557724821,-3.39038140719484,-1.08277623960184));
#9820=CARTESIAN_POINT('Ctrl Pts',(75.342557724821,-3.34615321126041,-1.18866045718896));
#9821=CARTESIAN_POINT('Ctrl Pts',(75.3425577248209,-3.29713139770849,-1.29231203608561));
#9822=CARTESIAN_POINT('Ctrl Pts',(75.3425577248209,-3.24352825182167,-1.39337011272125));
#9823=CARTESIAN_POINT('Ctrl Pts',(75.3425577248209,-3.19022134490429,-1.49386968966474));
#9824=CARTESIAN_POINT('Ctrl Pts',(75.3425577248209,-3.13238304795574,-1.59180509518516));
#9825=CARTESIAN_POINT('Ctrl Pts',(75.3425577248209,-3.07018008080428,-1.68679235709316));
#9826=CARTESIAN_POINT('Ctrl Pts',(75.3425577248209,-3.00962178257282,-1.7792681214857));
#9827=CARTESIAN_POINT('Ctrl Pts',(75.342557724821,-2.94492597991067,-1.86895010051926));
#9828=CARTESIAN_POINT('Ctrl Pts',(75.342557724821,-2.87621512332115,-1.95544730860172));
#9829=CARTESIAN_POINT('Ctrl Pts',(75.342557724821,-2.81023608483995,-2.03850554574002));
#9830=CARTESIAN_POINT('Ctrl Pts',(75.342557724821,-2.74055439650384,-2.11862751302659));
#9831=CARTESIAN_POINT('Ctrl Pts',(75.342557724821,-2.66725710276985,-2.19542711810058));
#9832=CARTESIAN_POINT('',(75.342557724821,-3.4544,-4.23041990297462E-16));
#9833=CARTESIAN_POINT('Origin',(75.342557724821,0.,0.));
#9834=CARTESIAN_POINT('Origin',(75.342557724821,0.,0.));
#9835=CARTESIAN_POINT('Ctrl Pts',(75.342557724821,-1.8872933839096,3.49128919534762));
#9836=CARTESIAN_POINT('Ctrl Pts',(75.3983874938273,-3.04449504617051,2.86573831175296));
#9837=CARTESIAN_POINT('Ctrl Pts',(75.5100470318401,-4.66829602391867,0.384128637822877));
#9838=CARTESIAN_POINT('Ctrl Pts',(75.6775363388591,-2.86406281752867,-3.71223393277672));
#9839=CARTESIAN_POINT('Ctrl Pts',(75.8450256458783,1.55028466462108,-4.42080615645044));
#9840=CARTESIAN_POINT('Ctrl Pts',(76.0125149528972,4.55194904417391,-1.11163115411373));
#9841=CARTESIAN_POINT('Ctrl Pts',(76.1800042599164,3.41272104871659,3.21148763121955));
#9842=CARTESIAN_POINT('Ctrl Pts',(76.3474935669354,-0.83234909652074,4.61115832194601));
#9843=CARTESIAN_POINT('Ctrl Pts',(76.5149828739545,-4.31977834004303,1.81565330639528));
#9844=CARTESIAN_POINT('Ctrl Pts',(76.6824721809736,-3.87667262829891,-2.63227689352042));
#9845=CARTESIAN_POINT('Ctrl Pts',(76.8499614879926,0.0939792462890116,-4.68487346091533));
#9846=CARTESIAN_POINT('Ctrl Pts',(77.0174507950118,3.9790823597631,-2.47467306941385));
#9847=CARTESIAN_POINT('Ctrl Pts',(77.1849401020308,4.24354045361218,1.98733341519075));
#9848=CARTESIAN_POINT('Ctrl Pts',(77.3524294090499,0.646690153391397,4.64099636386739));
#9849=CARTESIAN_POINT('Ctrl Pts',(77.519918716069,-3.53859451756145,3.07171589045833));
#9850=CARTESIAN_POINT('Ctrl Pts',(77.687408023088,-4.50402929941844,-1.29259812310088));
#9851=CARTESIAN_POINT('Ctrl Pts',(77.8548973301072,-1.3711384097138,-4.48074328527017));
#9852=CARTESIAN_POINT('Ctrl Pts',(78.0223866371261,3.00938367803536,-3.59175384599341));
#9853=CARTESIAN_POINT('Ctrl Pts',(78.1898759441454,4.65159553477052,0.565459445670238));
#9854=CARTESIAN_POINT('Ctrl Pts',(78.3573652511643,2.06120867216333,4.20814723864878));
#9855=CARTESIAN_POINT('Ctrl Pts',(78.5248545581835,-2.40472141992828,4.02174090914329));
#9856=CARTESIAN_POINT('Ctrl Pts',(78.6923438652025,-4.68253773972165,0.175855781190976));
#9857=CARTESIAN_POINT('Ctrl Pts',(78.8598331722217,-2.69960041692981,-3.83004470137668));
#9858=CARTESIAN_POINT('Ctrl Pts',(79.0273224792406,1.73976819338591,-4.35089548826393));
#9859=CARTESIAN_POINT('Ctrl Pts',(79.1948117862598,4.5960799186112,-0.912761895211113));
#9860=CARTESIAN_POINT('Ctrl Pts',(79.3623010932788,3.2703080678004,3.35591567615466));
#9861=CARTESIAN_POINT('Ctrl Pts',(79.529790400298,-1.03119568640402,4.57096492570699));
#9862=CARTESIAN_POINT('Ctrl Pts',(79.6972797073169,-4.39438970396336,1.62678333586707));
#9863=CARTESIAN_POINT('Ctrl Pts',(79.8647690143362,-3.75902292118467,-2.79764750621953));
#9864=CARTESIAN_POINT('Ctrl Pts',(80.032258321355,0.296769156290057,-4.67643164821721));
#9865=CARTESIAN_POINT('Ctrl Pts',(80.1997476283743,4.08252384642615,-2.30001824674852));
#9866=CARTESIAN_POINT('Ctrl Pts',(80.3672369353933,4.15349197522231,2.16923703262104));
#9867=CARTESIAN_POINT('Ctrl Pts',(80.5347262424123,0.445097936809096,4.66465140377808));
#9868=CARTESIAN_POINT('Ctrl Pts',(80.7022155494315,-3.66830141115372,2.91558735917221));
#9869=CARTESIAN_POINT('Ctrl Pts',(80.8697048564505,-4.44382514648826,-1.48643969251123));
#9870=CARTESIAN_POINT('Ctrl Pts',(81.0371941634697,-1.17580558461439,-4.53591954505886));
#9871=CARTESIAN_POINT('Ctrl Pts',(81.2046834704886,3.16210773630061,-3.45805719386958));
#9872=CARTESIAN_POINT('Ctrl Pts',(81.3721727775078,4.62274323446282,0.766374503930213));
#9873=CARTESIAN_POINT('Ctrl Pts',(81.5396620845268,1.87703356730924,4.29346362267612));
#9874=CARTESIAN_POINT('Ctrl Pts',(81.707151391546,-2.57663405263031,3.91382700829674));
#9875=CARTESIAN_POINT('Ctrl Pts',(81.874640698565,-4.68576042501116,-0.0270948601499234));
#9876=CARTESIAN_POINT('Ctrl Pts',(82.0421300055841,-2.53120077593259,-3.94336246418788));
#9877=CARTESIAN_POINT('Ctrl Pts',(82.2096193126032,1.92655929036014,-4.27146979303078));
#9878=CARTESIAN_POINT('Ctrl Pts',(82.3771086196222,4.63129675823398,-0.712864102910859));
#9879=CARTESIAN_POINT('Ctrl Pts',(82.5445979266413,3.12190600394933,3.49439376638532));
#9880=CARTESIAN_POINT('Ctrl Pts',(82.7120872336604,-1.22818205067104,4.52201876847685));
#9881=CARTESIAN_POINT('Ctrl Pts',(82.8795765406795,-4.46071774104712,1.43495021751798));
#9882=CARTESIAN_POINT('Ctrl Pts',(83.0470658476984,-3.63433915645072,-2.95781402186421));
#9883=CARTESIAN_POINT('Ctrl Pts',(83.2145551547178,0.499011969014512,-4.65919219895763));
#9884=CARTESIAN_POINT('Ctrl Pts',(83.3820444617366,4.17830011134652,-2.12105942197974));
#9885=CARTESIAN_POINT('Ctrl Pts',(83.5495337687558,4.05565256718464,2.34707629751062));
#9886=CARTESIAN_POINT('Ctrl Pts',(83.7170230757749,0.242669284494185,4.67955088768255));
#9887=CARTESIAN_POINT('Ctrl Pts',(83.8845123827939,-3.79112461211767,2.75398966364128));
#9888=CARTESIAN_POINT('Ctrl Pts',(84.0520016898132,-4.37528311379606,-1.6774929407239));
#9889=CARTESIAN_POINT('Ctrl Pts',(84.219490996832,-0.97826636104911,-4.58258440390215));
#9890=CARTESIAN_POINT('Ctrl Pts',(84.3869803038513,3.30889846384542,-3.31787218681023));
#9891=CARTESIAN_POINT('Ctrl Pts',(84.5544696108702,4.58521705524031,0.965851669968393));
#9892=CARTESIAN_POINT('Ctrl Pts',(84.7219589178894,1.68933645364314,4.37072388037037));
#9893=CARTESIAN_POINT('Ctrl Pts',(84.8894482249084,-2.74371198617596,3.79856939241103));
#9894=CARTESIAN_POINT('Ctrl Pts',(85.0569375319275,-4.68019095139554,-0.229994674987758));
#9895=CARTESIAN_POINT('Ctrl Pts',(85.2244268389466,-2.35805169304712,-4.04928106025811));
#9896=CARTESIAN_POINT('Ctrl Pts',(85.3919161459656,2.10973547078508,-4.18402929427589));
#9897=CARTESIAN_POINT('Ctrl Pts',(85.5594054529847,4.65782362744017,-0.511628720565475));
#9898=CARTESIAN_POINT('Ctrl Pts',(85.7268947600037,2.96764612613796,3.62631512172698));
#9899=CARTESIAN_POINT('Ctrl Pts',(85.894384067023,-1.42286390542218,4.46458768518373));
#9900=CARTESIAN_POINT('Ctrl Pts',(86.0618733740419,-4.5186758743998,1.24042461849348));
#9901=CARTESIAN_POINT('Ctrl Pts',(86.229362681061,-3.50283606998595,-3.11243061912276));
#9902=CARTESIAN_POINT('Ctrl Pts',(86.3968519880801,0.700318456568796,-4.63321043677455));
#9903=CARTESIAN_POINT('Ctrl Pts',(86.5643412950992,4.26623638905772,-1.93812073017321));
#9904=CARTESIAN_POINT('Ctrl Pts',(86.7318306021183,3.9502033026309,2.52051160678369));
#9905=CARTESIAN_POINT('Ctrl Pts',(86.8993199091373,0.0397852977070385,4.68566985842301));
#9906=CARTESIAN_POINT('Ctrl Pts',(87.0668092161565,-3.90683430574237,2.58722449731792));
#9907=CARTESIAN_POINT('Ctrl Pts',(87.2342985231754,-4.2985314832309,-1.86539861148232));
#9908=CARTESIAN_POINT('Ctrl Pts',(87.4017878301947,-0.778891559482246,-4.62065069342133));
#9909=CARTESIAN_POINT('Ctrl Pts',(87.5692771372135,3.44948051298471,-3.17146166342683));
#9910=CARTESIAN_POINT('Ctrl Pts',(87.7367664442328,4.53908736689592,1.16351655241039));
#9911=CARTESIAN_POINT('Ctrl Pts',(87.9042557512518,1.49846953985345,4.43978309494734));
#9912=CARTESIAN_POINT('Ctrl Pts',(88.071745058271,-2.90564173353642,3.67618430011031));
#9913=CARTESIAN_POINT('Ctrl Pts',(88.2392343652898,-4.66583976361946,-0.432462937455728));
#9914=CARTESIAN_POINT('Ctrl Pts',(88.4067236723092,-2.18047806078814,-4.1476017550482));
#9915=CARTESIAN_POINT('Ctrl Pts',(88.574212979328,2.28895303198969,-4.08873805829862));
#9916=CARTESIAN_POINT('Ctrl Pts',(88.7417022863472,4.67561075159403,-0.309433339534459));
#9917=CARTESIAN_POINT('Ctrl Pts',(88.9091915933663,2.80781788150847,3.75143221135632));
#9918=CARTESIAN_POINT('Ctrl Pts',(89.0766809003853,-1.614875957977,4.39877943664814));
#9919=CARTESIAN_POINT('Ctrl Pts',(89.2441702074045,-4.5681553537033,1.04357153872945));
#9920=CARTESIAN_POINT('Ctrl Pts',(89.4116595144236,-3.36476040873959,-3.26120718206482));
#9921=CARTESIAN_POINT('Ctrl Pts',(89.5791488214426,0.900310895961415,-4.59853511258327));
#9922=CARTESIAN_POINT('Ctrl Pts',(89.7466381284616,4.34616767952069,-1.75154543008276));
#9923=CARTESIAN_POINT('Ctrl Pts',(89.9141274354808,3.83734204230666,2.68921753416258));
#9924=CARTESIAN_POINT('Ctrl Pts',(90.0816167424998,-0.163173340857844,4.68299683371814));
#9925=CARTESIAN_POINT('Ctrl Pts',(90.2491060495189,-4.01521337859037,2.41560477313642));
#9926=CARTESIAN_POINT('Ctrl Pts',(90.416595356538,-4.21371426955079,-2.04980412993457));
#9927=CARTESIAN_POINT('Ctrl Pts',(90.584084663557,-0.578055276042246,-4.65004698078105));
#9928=CARTESIAN_POINT('Ctrl Pts',(90.7515739705762,3.58359009673503,-3.01910035578126));
#9929=CARTESIAN_POINT('Ctrl Pts',(90.9190632775952,4.48444073454358,1.35899828774903));
#9930=CARTESIAN_POINT('Ctrl Pts',(91.0865525846143,1.304790942286,4.5005116341675));
#9931=CARTESIAN_POINT('Ctrl Pts',(91.2540418916334,-3.06211942038283,3.54690147299146));
#9932=CARTESIAN_POINT('Ctrl Pts',(91.4215311986525,-4.64273386088492,-0.634119948295768));
#9933=CARTESIAN_POINT('Ctrl Pts',(91.5890205056715,-1.99881293045711,-4.2381396621777));
#9934=CARTESIAN_POINT('Ctrl Pts',(91.7565098126906,2.46387542085175,-3.98577567712814));
#9935=CARTESIAN_POINT('Ctrl Pts',(91.9239991197097,4.68462530132107,-0.10665579043167));
#9936=CARTESIAN_POINT('Ctrl Pts',(92.0914884267288,2.64272008949707,3.86950719504337));
#9937=CARTESIAN_POINT('Ctrl Pts',(92.2589777337479,-1.80385580473937,4.3247235657652));
#9938=CARTESIAN_POINT('Ctrl Pts',(92.4264670407669,-4.60906751720117,0.844748393393596));
#9939=CARTESIAN_POINT('Ctrl Pts',(92.593956347786,-3.22036301339166,-3.40384099298144));
#9940=CARTESIAN_POINT('Ctrl Pts',(92.761445654805,1.09859778933808,-4.55527773120639));
#9941=CARTESIAN_POINT('Ctrl Pts',(92.9289349618241,4.4179760167816,-1.56159205661129));
#9942=CARTESIAN_POINT('Ctrl Pts',(93.0964242688432,3.71721744660719,2.85269706473892));
#9943=CARTESIAN_POINT('Ctrl Pts',(93.2639135758623,-0.365701395163535,4.67189257704037));
#9944=CARTESIAN_POINT('Ctrl Pts',(93.4314028828815,-4.11630386768273,2.23875107871602));
#9945=CARTESIAN_POINT('Ctrl Pts',(93.5988921899004,-4.12050518287515,-2.22897883618675));
#9946=CARTESIAN_POINT('Ctrl Pts',(93.7663814969196,-0.377110979675515,-4.6734702206623));
#9947=CARTESIAN_POINT('Ctrl Pts',(93.9338708039386,3.71312449050035,-2.85538948225578));
#9948=CARTESIAN_POINT('Ctrl Pts',(94.0455303419513,4.18043603275127,0.073217031354101));
#9949=CARTESIAN_POINT('Ctrl Pts',(94.1013601109577,3.74476191969682,1.31443323424532));
#9950=CARTESIAN_POINT('Ctrl Pts',(75.2435710211684,-1.8057623097247,3.34046550210861));
#9951=CARTESIAN_POINT('Ctrl Pts',(75.2994007901748,-2.91297286017594,2.74193841668523));
#9952=CARTESIAN_POINT('Ctrl Pts',(75.4110603281875,-4.46662563568538,0.367534280668929));
#9953=CARTESIAN_POINT('Ctrl Pts',(75.5785496352065,-2.74033530381143,-3.55186542688076));
#9954=CARTESIAN_POINT('Ctrl Pts',(75.7460389422257,1.48331236710945,-4.22982733049178));
#9955=CARTESIAN_POINT('Ctrl Pts',(75.9135282492446,4.35530484546559,-1.06360868825602));
#9956=CARTESIAN_POINT('Ctrl Pts',(76.0810175562638,3.26529149941203,3.07275136555087));
#9957=CARTESIAN_POINT('Ctrl Pts',(76.2485068632828,-0.796391615551045,4.41195628243795));
#9958=CARTESIAN_POINT('Ctrl Pts',(76.415996170302,-4.13316391575316,1.73721708355901));
#9959=CARTESIAN_POINT('Ctrl Pts',(76.5834854773211,-3.7092003707564,-2.51856253172034));
#9960=CARTESIAN_POINT('Ctrl Pts',(76.7509747843401,0.0899193428493282,-4.48248692740379));
#9961=CARTESIAN_POINT('Ctrl Pts',(76.9184640913591,3.80718600182134,-2.36776719281517));
#9962=CARTESIAN_POINT('Ctrl Pts',(77.0859533983784,4.06021950601614,1.90148061165451));
#9963=CARTESIAN_POINT('Ctrl Pts',(77.2534427053972,0.618753138764886,4.44050532094832));
#9964=CARTESIAN_POINT('Ctrl Pts',(77.4209320124165,-3.38572723440279,2.93901776399053));
#9965=CARTESIAN_POINT('Ctrl Pts',(77.5884213194354,-4.30945523368357,-1.23675788418292));
#9966=CARTESIAN_POINT('Ctrl Pts',(77.7559106264547,-1.31190523041416,-4.28717517534649));
#9967=CARTESIAN_POINT('Ctrl Pts',(77.9233999334736,2.87937830314423,-3.4365900798465));
#9968=CARTESIAN_POINT('Ctrl Pts',(78.0908892404928,4.45064660766843,0.541031597617288));
#9969=CARTESIAN_POINT('Ctrl Pts',(78.2583785475117,1.97216445752588,4.02635527793915));
#9970=CARTESIAN_POINT('Ctrl Pts',(78.425867854531,-2.30083745458738,3.8480017018683));
#9971=CARTESIAN_POINT('Ctrl Pts',(78.5933571615498,-4.48025210936568,0.168258811443526));
#9972=CARTESIAN_POINT('Ctrl Pts',(78.7608464685692,-2.58297767891845,-3.66458677027721));
#9973=CARTESIAN_POINT('Ctrl Pts',(78.928335775588,1.66461020743164,-4.16293680317093));
#9974=CARTESIAN_POINT('Ctrl Pts',(79.0958250826073,4.3975292661272,-0.873330581337993));
#9975=CARTESIAN_POINT('Ctrl Pts',(79.2633143896262,3.12903075927143,3.21094011894477));
#9976=CARTESIAN_POINT('Ctrl Pts',(79.4308036966454,-0.986648032751362,4.37349924091645));
#9977=CARTESIAN_POINT('Ctrl Pts',(79.5982930036644,-4.20455206875214,1.55650629575761));
#9978=CARTESIAN_POINT('Ctrl Pts',(79.7657823106836,-3.59663313098949,-2.67678913395085));
#9979=CARTESIAN_POINT('Ctrl Pts',(79.9332716177025,0.283948728738327,-4.47440980101422));
#9980=CARTESIAN_POINT('Ctrl Pts',(80.1007609247218,3.90615881626054,-2.20065745848898));
#9981=CARTESIAN_POINT('Ctrl Pts',(80.2682502317407,3.9740611218927,2.07552599281181));
#9982=CARTESIAN_POINT('Ctrl Pts',(80.4357395387598,0.425869705938943,4.46313846313487));
#9983=CARTESIAN_POINT('Ctrl Pts',(80.6032288457789,-3.50983079019188,2.78963398525597));
#9984=CARTESIAN_POINT('Ctrl Pts',(80.770718152798,-4.25185190015997,-1.42222549779475));
#9985=CARTESIAN_POINT('Ctrl Pts',(80.9382074598171,-1.12501078335905,-4.33996782071231));
#9986=CARTESIAN_POINT('Ctrl Pts',(81.1056967668361,3.02550468209242,-3.30866912309442));
#9987=CARTESIAN_POINT('Ctrl Pts',(81.2731860738552,4.42304072673403,0.733267125360433));
#9988=CARTESIAN_POINT('Ctrl Pts',(81.4406753808743,1.79594571720148,4.10798599417651));
#9989=CARTESIAN_POINT('Ctrl Pts',(81.6081646878934,-2.46532346155667,3.74474968153832));
#9990=CARTESIAN_POINT('Ctrl Pts',(81.7756539949124,-4.48333557465068,-0.0259243621914455));
#9991=CARTESIAN_POINT('Ctrl Pts',(81.9431433019315,-2.4218529024123,-3.77300920573496));
#9992=CARTESIAN_POINT('Ctrl Pts',(82.1106326089505,1.84333192901658,-4.08694229797184));
#9993=CARTESIAN_POINT('Ctrl Pts',(82.2781219159698,4.43122473827827,-0.682068373665113));
#9994=CARTESIAN_POINT('Ctrl Pts',(82.4456112229886,2.98703966457872,3.34343595567747));
#9995=CARTESIAN_POINT('Ctrl Pts',(82.613100530008,-1.17512458608205,4.32666755767865));
#9996=CARTESIAN_POINT('Ctrl Pts',(82.7805898370269,-4.26801473463389,1.3729603681212));
#9997=CARTESIAN_POINT('Ctrl Pts',(82.948079144046,-3.47733570489205,-2.83003645611967));
#9998=CARTESIAN_POINT('Ctrl Pts',(83.1155684510651,0.477454651953081,-4.45791509596267));
#9999=CARTESIAN_POINT('Ctrl Pts',(83.2830577580841,3.99779754653636,-2.02942965495022));
#10000=CARTESIAN_POINT('Ctrl Pts',(83.4505470651032,3.88044837628226,2.24568260145816));
#10001=CARTESIAN_POINT('Ctrl Pts',(83.6180363721223,0.232185971404038,4.47739428933466));
#10002=CARTESIAN_POINT('Ctrl Pts',(83.7855256791413,-3.62734802887419,2.63501731017198));
#10003=CARTESIAN_POINT('Ctrl Pts',(83.9530149861606,-4.18627088328007,-1.60502524568462));
#10004=CARTESIAN_POINT('Ctrl Pts',(84.1205042931794,-0.936005254251792,
-4.38461675765357));
#10005=CARTESIAN_POINT('Ctrl Pts',(84.2879936001987,3.1659540502073,-3.17454010834003));
#10006=CARTESIAN_POINT('Ctrl Pts',(84.4554829072177,4.38713567845393,0.924126877825758));
#10007=CARTESIAN_POINT('Ctrl Pts',(84.6229722142368,1.61635711884576,4.18190860873838));
#10008=CARTESIAN_POINT('Ctrl Pts',(84.7904615212559,-2.62518362837316,3.63447119465887));
#10009=CARTESIAN_POINT('Ctrl Pts',(84.9579508282749,-4.47800670229525,-0.220058905028287));
#10010=CARTESIAN_POINT('Ctrl Pts',(85.125440135294,-2.25618385990748,-3.87435211845496));
#10011=CARTESIAN_POINT('Ctrl Pts',(85.2929294423131,2.01859489844716,-4.00327922876317));
#10012=CARTESIAN_POINT('Ctrl Pts',(85.4604187493321,4.45660564673476,-0.489526359837044));
#10013=CARTESIAN_POINT('Ctrl Pts',(85.6279080563512,2.83944381348879,3.46965830846837));
#10014=CARTESIAN_POINT('Ctrl Pts',(85.7953973633703,-1.36139618470794,4.2717174971838));
#10015=CARTESIAN_POINT('Ctrl Pts',(85.9628866703895,-4.32346907662573,1.18683827497456));
#10016=CARTESIAN_POINT('Ctrl Pts',(86.1303759774084,-3.35151355176255,-2.97797361637666));
#10017=CARTESIAN_POINT('Ctrl Pts',(86.2978652844277,0.67006469924502,-4.43305574590589));
#10018=CARTESIAN_POINT('Ctrl Pts',(86.4653545914465,4.08193497705043,-1.85439391462973));
#10019=CARTESIAN_POINT('Ctrl Pts',(86.6328438984658,3.77955451995724,2.41162550537063));
#10020=CARTESIAN_POINT('Ctrl Pts',(86.8003332054847,0.0380665728460967,
4.48324892053913));
#10021=CARTESIAN_POINT('Ctrl Pts',(86.9678225125039,-3.7380590637343,2.47545639903379));
#10022=CARTESIAN_POINT('Ctrl Pts',(87.135311819523,-4.11283492315532,-1.78481339146628));
#10023=CARTESIAN_POINT('Ctrl Pts',(87.3028011265419,-0.745243444112614,
-4.42103858346553));
#10024=CARTESIAN_POINT('Ctrl Pts',(87.4702904335612,3.30046295482377,-3.03445451956679));
#10025=CARTESIAN_POINT('Ctrl Pts',(87.63777974058,4.34299879264601,1.11325263734626));
#10026=CARTESIAN_POINT('Ctrl Pts',(87.8052690475994,1.43373565573179,4.24798446524562));
#10027=CARTESIAN_POINT('Ctrl Pts',(87.9727583546183,-2.78011801064765,3.51737313834554));
#10028=CARTESIAN_POINT('Ctrl Pts',(88.1402476616373,-4.46427548583109,-0.413780538557639));
#10029=CARTESIAN_POINT('Ctrl Pts',(88.3077369686566,-2.08628140856209,-3.96842535923012));
#10030=CARTESIAN_POINT('Ctrl Pts',(88.4752262756754,2.19007026100774,-3.91210457418012));
#10031=CARTESIAN_POINT('Ctrl Pts',(88.6427155826948,4.47362436712517,-0.296065819266569));
#10032=CARTESIAN_POINT('Ctrl Pts',(88.8102048897136,2.68652014902731,3.58937033982573));
#10033=CARTESIAN_POINT('Ctrl Pts',(88.9776941967329,-1.54511331659239,4.20875216498494));
#10034=CARTESIAN_POINT('Ctrl Pts',(89.1451835037518,-4.37081104242332,0.998489248256337));
#10035=CARTESIAN_POINT('Ctrl Pts',(89.3126728107711,-3.21940275908204,-3.12032303179962));
#10036=CARTESIAN_POINT('Ctrl Pts',(89.4801621177899,0.86141746525588,-4.39987839571967));
#10037=CARTESIAN_POINT('Ctrl Pts',(89.6476514248092,4.1584132357654,-1.67587866750318));
#10038=CARTESIAN_POINT('Ctrl Pts',(89.8151407318281,3.67156886607901,2.57304333668676));
#10039=CARTESIAN_POINT('Ctrl Pts',(89.9826300388473,-0.156124252532783,
4.48069137050152));
#10040=CARTESIAN_POINT('Ctrl Pts',(90.1501193458663,-3.84175616063527,2.31125064693693));
#10041=CARTESIAN_POINT('Ctrl Pts',(90.3176086528854,-4.0316818131062,-1.9612525915214));
#10042=CARTESIAN_POINT('Ctrl Pts',(90.4850979599046,-0.553083288117217,
-4.4491649512113));
#10043=CARTESIAN_POINT('Ctrl Pts',(90.6525872669235,3.42877900455607,-2.88867522041151));
#10044=CARTESIAN_POINT('Ctrl Pts',(90.8200765739428,4.2907128948113,1.30028956171827));
#10045=CARTESIAN_POINT('Ctrl Pts',(90.9875658809616,1.24842397357924,4.30608953157147));
#10046=CARTESIAN_POINT('Ctrl Pts',(91.1550551879809,-2.92983586142229,3.39367532935823));
#10047=CARTESIAN_POINT('Ctrl Pts',(91.3225444949997,-4.4421677580947,-0.606725966529394));
#10048=CARTESIAN_POINT('Ctrl Pts',(91.4900338020191,-1.91246421186136,-4.05505202877162));
#10049=CARTESIAN_POINT('Ctrl Pts',(91.657523109038,2.35743600267096,-3.81359016787621));
#10050=CARTESIAN_POINT('Ctrl Pts',(91.825012416057,4.482249488304,-0.102048260285022));
#10051=CARTESIAN_POINT('Ctrl Pts',(91.9925017230764,2.5285545816308,3.7023444842175));
#10052=CARTESIAN_POINT('Ctrl Pts',(92.1599910300952,-1.72592923397463,4.13789550772414));
#10053=CARTESIAN_POINT('Ctrl Pts',(92.3274803371144,-4.40995580045808,0.808255262798993));
#10054=CARTESIAN_POINT('Ctrl Pts',(92.4949696441334,-3.08124333121314,-3.25679506208464));
#10055=CARTESIAN_POINT('Ctrl Pts',(92.6624589511525,1.05113836483867,-4.35848973321828));
#10056=CARTESIAN_POINT('Ctrl Pts',(92.8299482581715,4.22711945285663,-1.49413127976568));
#10057=CARTESIAN_POINT('Ctrl Pts',(92.9974375651909,3.55663365291376,2.7294605515422));
#10058=CARTESIAN_POINT('Ctrl Pts',(93.1649268722096,-0.349903094892468,
4.47006681771222));
#10059=CARTESIAN_POINT('Ctrl Pts',(93.3324161792289,-3.93847954059884,2.14203703211549));
#10060=CARTESIAN_POINT('Ctrl Pts',(93.4999054862479,-3.94249935897495,-2.13268695046349));
#10061=CARTESIAN_POINT('Ctrl Pts',(93.667394793267,-0.360819785353534,-4.47157630712969));
#10062=CARTESIAN_POINT('Ctrl Pts',(93.834884100286,3.55271751251074,-2.73203665662233));
#10063=CARTESIAN_POINT('Ctrl Pts',(93.9465436382988,3.99984119613641,0.0700540555996051));
#10064=CARTESIAN_POINT('Ctrl Pts',(94.0023734073051,3.58298820476592,1.25764971852592));
#10065=CARTESIAN_POINT('Ctrl Pts',(75.1445843175159,-1.72423123553981,3.18964180886959));
#10066=CARTESIAN_POINT('Ctrl Pts',(75.2004140865222,-2.78145067418138,2.6181385216175));
#10067=CARTESIAN_POINT('Ctrl Pts',(75.312073624535,-4.26495524745209,0.35093992351498));
#10068=CARTESIAN_POINT('Ctrl Pts',(75.4795629315539,-2.6166077900942,-3.39149692098481));
#10069=CARTESIAN_POINT('Ctrl Pts',(75.6470522385733,1.41634006959782,-4.03884850453312));
#10070=CARTESIAN_POINT('Ctrl Pts',(75.814541545592,4.15866064675728,-1.0155862223983));
#10071=CARTESIAN_POINT('Ctrl Pts',(75.9820308526114,3.11786195010748,2.93401509988218));
#10072=CARTESIAN_POINT('Ctrl Pts',(76.1495201596302,-0.760434134581352,
4.21275424292987));
#10073=CARTESIAN_POINT('Ctrl Pts',(76.3170094666494,-3.9465494914633,1.65878086072273));
#10074=CARTESIAN_POINT('Ctrl Pts',(76.4844987736685,-3.54172811321389,-2.40484816992026));
#10075=CARTESIAN_POINT('Ctrl Pts',(76.6519880806875,0.0858594394096438,
-4.28010039389224));
#10076=CARTESIAN_POINT('Ctrl Pts',(76.8194773877067,3.63528964387957,-2.26086131621649));
#10077=CARTESIAN_POINT('Ctrl Pts',(76.9869666947257,3.87689855842009,1.81562780811827));
#10078=CARTESIAN_POINT('Ctrl Pts',(77.1544560017448,0.590816124138375,4.24001427802925));
#10079=CARTESIAN_POINT('Ctrl Pts',(77.3219453087639,-3.23285995124413,2.80631963752273));
#10080=CARTESIAN_POINT('Ctrl Pts',(77.4894346157829,-4.1148811679487,-1.18091764526496));
#10081=CARTESIAN_POINT('Ctrl Pts',(77.6569239228021,-1.25267205111452,-4.09360706542282));
#10082=CARTESIAN_POINT('Ctrl Pts',(77.8244132298211,2.7493729282531,-3.28142631369958));
#10083=CARTESIAN_POINT('Ctrl Pts',(77.9919025368402,4.24969768056634,0.516603749564329));
#10084=CARTESIAN_POINT('Ctrl Pts',(78.1593918438592,1.88312024288842,3.84456331722953));
#10085=CARTESIAN_POINT('Ctrl Pts',(78.3268811508785,-2.19695348924648,3.67426249459331));
#10086=CARTESIAN_POINT('Ctrl Pts',(78.4943704578973,-4.2779664790097,0.160661841696076));
#10087=CARTESIAN_POINT('Ctrl Pts',(78.6618597649166,-2.46635494090708,-3.49912883917774));
#10088=CARTESIAN_POINT('Ctrl Pts',(78.8293490719354,1.58945222147737,-3.97497811807793));
#10089=CARTESIAN_POINT('Ctrl Pts',(78.9968383789548,4.19897861364319,-0.833899267464873));
#10090=CARTESIAN_POINT('Ctrl Pts',(79.1643276859736,2.98775345074245,3.06596456173489));
#10091=CARTESIAN_POINT('Ctrl Pts',(79.3318169929929,-0.94210037909871,4.17603355612591));
#10092=CARTESIAN_POINT('Ctrl Pts',(79.4993063000118,-4.01471443354093,1.48622925564816));
#10093=CARTESIAN_POINT('Ctrl Pts',(79.6667956070311,-3.43424334079431,-2.55593076168216));
#10094=CARTESIAN_POINT('Ctrl Pts',(79.8342849140499,0.271128301186596,-4.27238795381124));
#10095=CARTESIAN_POINT('Ctrl Pts',(80.0017742210692,3.72979378609493,-2.10129667022944));
#10096=CARTESIAN_POINT('Ctrl Pts',(80.1692635280881,3.7946302685631,1.98181495300258));
#10097=CARTESIAN_POINT('Ctrl Pts',(80.3367528351073,0.406641475068789,4.26162552249166));
#10098=CARTESIAN_POINT('Ctrl Pts',(80.5042421421263,-3.35136016923003,2.66368061133973));
#10099=CARTESIAN_POINT('Ctrl Pts',(80.6717314491454,-4.05987865383168,-1.35801130307826));
#10100=CARTESIAN_POINT('Ctrl Pts',(80.8392207561645,-1.07421598210371,-4.14401609636577));
#10101=CARTESIAN_POINT('Ctrl Pts',(81.0067100631835,2.88890162788424,-3.15928105231925));
#10102=CARTESIAN_POINT('Ctrl Pts',(81.1741993702027,4.22333821900523,0.700159746790646));
#10103=CARTESIAN_POINT('Ctrl Pts',(81.3416886772216,1.71485786709373,3.9225083656769));
#10104=CARTESIAN_POINT('Ctrl Pts',(81.5091779842409,-2.35401287048305,3.5756723547799));
#10105=CARTESIAN_POINT('Ctrl Pts',(81.6766672912598,-4.28091072429019,-0.0247538642329713));
#10106=CARTESIAN_POINT('Ctrl Pts',(81.844156598279,-2.31250502889201,-3.60265594728204));
#10107=CARTESIAN_POINT('Ctrl Pts',(82.0116459052979,1.76010456767303,-3.90241480291292));
#10108=CARTESIAN_POINT('Ctrl Pts',(82.1791352123172,4.23115271832256,-0.651272644419364));
#10109=CARTESIAN_POINT('Ctrl Pts',(82.3466245193362,2.85217332520811,3.19247814496963));
#10110=CARTESIAN_POINT('Ctrl Pts',(82.5141138263553,-1.12206712149307,4.13131634688045));
#10111=CARTESIAN_POINT('Ctrl Pts',(82.6816031333744,-4.07531172822065,1.31097051872443));
#10112=CARTESIAN_POINT('Ctrl Pts',(82.8490924403933,-3.32033225333338,-2.70225889037514));
#10113=CARTESIAN_POINT('Ctrl Pts',(83.0165817474127,0.455897334891659,-4.2566379929677));
#10114=CARTESIAN_POINT('Ctrl Pts',(83.1840710544314,3.81729498172618,-1.93779988792069));
#10115=CARTESIAN_POINT('Ctrl Pts',(83.3515603614509,3.70524418537989,2.1442889054057));
#10116=CARTESIAN_POINT('Ctrl Pts',(83.5190496684696,0.221702658313887,4.27523769098678));
#10117=CARTESIAN_POINT('Ctrl Pts',(83.6865389754889,-3.4635714456307,2.51604495670267));
#10118=CARTESIAN_POINT('Ctrl Pts',(83.8540282825079,-3.99725865276408,-1.53255755064535));
#10119=CARTESIAN_POINT('Ctrl Pts',(84.0215175895269,-0.893744147454468,
-4.186649111405));
#10120=CARTESIAN_POINT('Ctrl Pts',(84.1890068965461,3.02300963656918,-3.03120802986982));
#10121=CARTESIAN_POINT('Ctrl Pts',(84.3564962035651,4.18905430166755,0.882402085683122));
#10122=CARTESIAN_POINT('Ctrl Pts',(84.5239855105842,1.54337778404837,3.99309333710638));
#10123=CARTESIAN_POINT('Ctrl Pts',(84.6914748176033,-2.50665527057035,3.47037299690671));
#10124=CARTESIAN_POINT('Ctrl Pts',(84.8589641246224,-4.27582245319496,-0.210123135068815));
#10125=CARTESIAN_POINT('Ctrl Pts',(85.0264534316414,-2.15431602676784,-3.69942317665181));
#10126=CARTESIAN_POINT('Ctrl Pts',(85.1939427386606,1.92745432610924,-3.82252916325045));
#10127=CARTESIAN_POINT('Ctrl Pts',(85.3614320456795,4.25538766602934,-0.467423999108614));
#10128=CARTESIAN_POINT('Ctrl Pts',(85.5289213526986,2.71124150083964,3.31300149520976));
#10129=CARTESIAN_POINT('Ctrl Pts',(85.6964106597178,-1.2999284639937,4.07884730918386));
#10130=CARTESIAN_POINT('Ctrl Pts',(85.8638999667367,-4.12826227885166,1.13325193145564));
#10131=CARTESIAN_POINT('Ctrl Pts',(86.031389273756,-3.20019103353916,-2.84351661363055));
#10132=CARTESIAN_POINT('Ctrl Pts',(86.1988785807749,0.63981094192125,-4.23290105503723));
#10133=CARTESIAN_POINT('Ctrl Pts',(86.3663678877942,3.89763356504313,-1.77066709908625));
#10134=CARTESIAN_POINT('Ctrl Pts',(86.5338571948131,3.60890573728359,2.30273940395758));
#10135=CARTESIAN_POINT('Ctrl Pts',(86.7013465018323,0.0363478479851531,
4.28082798265526));
#10136=CARTESIAN_POINT('Ctrl Pts',(86.8688358088512,-3.56928382172623,2.36368830074965));
#10137=CARTESIAN_POINT('Ctrl Pts',(87.0363251158705,-3.92713836307975,-1.70422817145024));
#10138=CARTESIAN_POINT('Ctrl Pts',(87.2038144228895,-0.71159532874298,-4.22142647350973));
#10139=CARTESIAN_POINT('Ctrl Pts',(87.3713037299085,3.15144539666283,-2.89744737570675));
#10140=CARTESIAN_POINT('Ctrl Pts',(87.5387930369278,4.14691021839611,1.06298872228213));
#10141=CARTESIAN_POINT('Ctrl Pts',(87.7062823439466,1.36900177161012,4.05618583554389));
#10142=CARTESIAN_POINT('Ctrl Pts',(87.8737716509658,-2.65459428775888,3.35856197658078));
#10143=CARTESIAN_POINT('Ctrl Pts',(88.0412609579848,-4.26271120804273,-0.39509813965955));
#10144=CARTESIAN_POINT('Ctrl Pts',(88.208750265004,-1.99208475633604,-3.78924896341204));
#10145=CARTESIAN_POINT('Ctrl Pts',(88.3762395720229,2.09118749002578,-3.73547109006162));
#10146=CARTESIAN_POINT('Ctrl Pts',(88.5437288790422,4.2716379826563,-0.282698298998683));
#10147=CARTESIAN_POINT('Ctrl Pts',(88.7112181860611,2.56522241654614,3.42730846829514));
#10148=CARTESIAN_POINT('Ctrl Pts',(88.8787074930802,-1.47535067520778,4.01872489332174));
#10149=CARTESIAN_POINT('Ctrl Pts',(89.0461968000995,-4.17346673114334,0.953406957783226));
#10150=CARTESIAN_POINT('Ctrl Pts',(89.2136861071183,-3.07404510942449,-2.97943888153443));
#10151=CARTESIAN_POINT('Ctrl Pts',(89.3811754141374,0.822524034550345,-4.20122167885608));
#10152=CARTESIAN_POINT('Ctrl Pts',(89.5486647211566,3.97065879201011,-1.60021190492361));
#10153=CARTESIAN_POINT('Ctrl Pts',(89.7161540281756,3.50579568985136,2.45686913921093));
#10154=CARTESIAN_POINT('Ctrl Pts',(89.8836433351946,-0.149075164207724,
4.2783859072849));
#10155=CARTESIAN_POINT('Ctrl Pts',(90.0511326422139,-3.66829894268017,2.20689652073743));
#10156=CARTESIAN_POINT('Ctrl Pts',(90.2186219492327,-3.8496493566616,-1.87270105310823));
#10157=CARTESIAN_POINT('Ctrl Pts',(90.3861112562521,-0.528111300192195,
-4.24828292164156));
#10158=CARTESIAN_POINT('Ctrl Pts',(90.5536005632709,3.27396791237712,-2.75825008504176));
#10159=CARTESIAN_POINT('Ctrl Pts',(90.7210898702902,4.09698505507901,1.24158083568751));
#10160=CARTESIAN_POINT('Ctrl Pts',(90.888579177309,1.19205700487249,4.11166742897543));
#10161=CARTESIAN_POINT('Ctrl Pts',(91.0560684843284,-2.79755230246175,3.240449185725));
#10162=CARTESIAN_POINT('Ctrl Pts',(91.2235577913473,-4.24160165530447,-0.579331984763014));
#10163=CARTESIAN_POINT('Ctrl Pts',(91.3910470983663,-1.82611549326562,-3.87196439536554));
#10164=CARTESIAN_POINT('Ctrl Pts',(91.5585364053856,2.25099658449016,-3.64140465862427));
#10165=CARTESIAN_POINT('Ctrl Pts',(91.7260257124045,4.27987367528693,-0.0974407301383736));
#10166=CARTESIAN_POINT('Ctrl Pts',(91.8935150194238,2.41438907376452,3.53518177339162));
#10167=CARTESIAN_POINT('Ctrl Pts',(92.0610043264426,-1.64800266320989,3.95106744968309));
#10168=CARTESIAN_POINT('Ctrl Pts',(92.2284936334618,-4.21084408371499,0.771762132204391));
#10169=CARTESIAN_POINT('Ctrl Pts',(92.3959829404809,-2.94212364903462,-3.10974913118785));
#10170=CARTESIAN_POINT('Ctrl Pts',(92.5634722474998,1.00367894033927,-4.16170173523016));
#10171=CARTESIAN_POINT('Ctrl Pts',(92.7309615545192,4.03626288893166,-1.42667050292008));
#10172=CARTESIAN_POINT('Ctrl Pts',(92.8984508615381,3.39604985922033,2.60622403834548));
#10173=CARTESIAN_POINT('Ctrl Pts',(93.0659401685572,-0.334104794621406,
4.26824105838408));
#10174=CARTESIAN_POINT('Ctrl Pts',(93.2334294755763,-3.76065521351494,2.04532298551495));
#10175=CARTESIAN_POINT('Ctrl Pts',(93.4009187825955,-3.76449353507474,-2.03639506474021));
#10176=CARTESIAN_POINT('Ctrl Pts',(93.5684080896143,-0.344528591031553,
-4.26968239359708));
#10177=CARTESIAN_POINT('Ctrl Pts',(93.7358973966336,3.39231053452112,-2.60868383098888));
#10178=CARTESIAN_POINT('Ctrl Pts',(93.8475569346462,3.81924635952156,0.0668910798451053));
#10179=CARTESIAN_POINT('Ctrl Pts',(93.9033867036526,3.42121448983501,1.20086620280652));
#10180=CARTESIAN_POINT('Ctrl Pts',(75.0455976138633,-1.64270016135492,3.03881811563057));
#10181=CARTESIAN_POINT('Ctrl Pts',(75.1014273828696,-2.64992848818681,2.49433862654978));
#10182=CARTESIAN_POINT('Ctrl Pts',(75.2130869208824,-4.06328485921881,0.334345566361032));
#10183=CARTESIAN_POINT('Ctrl Pts',(75.3805762279014,-2.49288027637696,-3.23112841508885));
#10184=CARTESIAN_POINT('Ctrl Pts',(75.5480655349206,1.34936777208619,-3.84786967857446));
#10185=CARTESIAN_POINT('Ctrl Pts',(75.7155548419395,3.96201644804897,-0.96756375654059));
#10186=CARTESIAN_POINT('Ctrl Pts',(75.8830441489588,2.97043240080292,2.7952788342135));
#10187=CARTESIAN_POINT('Ctrl Pts',(76.0505334559776,-0.724476653611653,
4.01355220342181));
#10188=CARTESIAN_POINT('Ctrl Pts',(76.2180227629969,-3.75993506717345,1.58034463788646));
#10189=CARTESIAN_POINT('Ctrl Pts',(76.3855120700159,-3.37425585567137,-2.29113380812018));
#10190=CARTESIAN_POINT('Ctrl Pts',(76.553001377035,0.0817995359699572,-4.0777138603807));
#10191=CARTESIAN_POINT('Ctrl Pts',(76.7204906840541,3.4633932859378,-2.15395543961782));
#10192=CARTESIAN_POINT('Ctrl Pts',(76.8879799910732,3.69357761082405,1.72977500458203));
#10193=CARTESIAN_POINT('Ctrl Pts',(77.0554692980922,0.562879109511871,4.03952323511018));
#10194=CARTESIAN_POINT('Ctrl Pts',(77.2229586051114,-3.07999266808548,2.67362151105493));
#10195=CARTESIAN_POINT('Ctrl Pts',(77.3904479121303,-3.92030710221381,-1.12507740634701));
#10196=CARTESIAN_POINT('Ctrl Pts',(77.5579372191495,-1.19343887181489,-3.90003895549915));
#10197=CARTESIAN_POINT('Ctrl Pts',(77.7254265261685,2.61936755336198,-3.12626254755267));
#10198=CARTESIAN_POINT('Ctrl Pts',(77.8929158331876,4.04874875346425,0.492175901511377));
#10199=CARTESIAN_POINT('Ctrl Pts',(78.0604051402066,1.79407602825097,3.6627713565199));
#10200=CARTESIAN_POINT('Ctrl Pts',(78.2278944472258,-2.09306952390558,3.50052328731832));
#10201=CARTESIAN_POINT('Ctrl Pts',(78.3953837542448,-4.07568084865373,0.153064871948625));
#10202=CARTESIAN_POINT('Ctrl Pts',(78.562873061264,-2.34973220289571,-3.33367090807826));
#10203=CARTESIAN_POINT('Ctrl Pts',(78.730362368283,1.5142942355231,-3.78701943298493));
#10204=CARTESIAN_POINT('Ctrl Pts',(78.8978516753021,4.00042796115919,-0.794467953591753));
#10205=CARTESIAN_POINT('Ctrl Pts',(79.0653409823211,2.84647614221347,2.92098900452501));
#10206=CARTESIAN_POINT('Ctrl Pts',(79.2328302893403,-0.897552725446056,
3.97856787133537));
#10207=CARTESIAN_POINT('Ctrl Pts',(79.4003195963593,-3.82487679832971,1.4159522155387));
#10208=CARTESIAN_POINT('Ctrl Pts',(79.5678089033784,-3.27185355059914,-2.43507238941348));
#10209=CARTESIAN_POINT('Ctrl Pts',(79.7352982103974,0.258307873634867,-4.07036610660826));
#10210=CARTESIAN_POINT('Ctrl Pts',(79.9027875174166,3.55342875592932,-2.00193588196991));
#10211=CARTESIAN_POINT('Ctrl Pts',(80.0702768244356,3.6151994152335,1.88810391319336));
#10212=CARTESIAN_POINT('Ctrl Pts',(80.2377661314546,0.387413244198636,4.06011258184844));
#10213=CARTESIAN_POINT('Ctrl Pts',(80.4052554384739,-3.19288954826819,2.53772723742349));
#10214=CARTESIAN_POINT('Ctrl Pts',(80.5727447454928,-3.86790540750339,-1.29379710836178));
#10215=CARTESIAN_POINT('Ctrl Pts',(80.740234052512,-1.02342118084837,-3.94806437201922));
#10216=CARTESIAN_POINT('Ctrl Pts',(80.907723359531,2.75229857367605,-3.00989298154409));
#10217=CARTESIAN_POINT('Ctrl Pts',(81.0752126665501,4.02363571127644,0.667052368220863));
#10218=CARTESIAN_POINT('Ctrl Pts',(81.2427019735692,1.63377001698596,3.73703073717729));
#10219=CARTESIAN_POINT('Ctrl Pts',(81.4101912805883,-2.24270227940942,3.40659502802148));
#10220=CARTESIAN_POINT('Ctrl Pts',(81.5776805876073,-4.07848587392971,-0.0235833662744953));
#10221=CARTESIAN_POINT('Ctrl Pts',(81.7451698946264,-2.20315715537172,-3.43230268882913));
#10222=CARTESIAN_POINT('Ctrl Pts',(81.9126592016455,1.67687720632947,-3.71788730785399));
#10223=CARTESIAN_POINT('Ctrl Pts',(82.0801485086645,4.03108069836686,-0.620476915173612));
#10224=CARTESIAN_POINT('Ctrl Pts',(82.2476378156836,2.7173069858375,3.04152033426178));
#10225=CARTESIAN_POINT('Ctrl Pts',(82.4151271227027,-1.06900965690408,3.93596513608225));
#10226=CARTESIAN_POINT('Ctrl Pts',(82.5826164297217,-3.88260872180742,1.24898066932765));
#10227=CARTESIAN_POINT('Ctrl Pts',(82.7501057367409,-3.1633288017747,-2.5744813246306));
#10228=CARTESIAN_POINT('Ctrl Pts',(82.9175950437599,0.434340017830227,-4.05536088997273));
#10229=CARTESIAN_POINT('Ctrl Pts',(83.0850843507791,3.63679241691602,-1.84617012089117));
#10230=CARTESIAN_POINT('Ctrl Pts',(83.252573657798,3.53003999447751,2.04289520935324));
#10231=CARTESIAN_POINT('Ctrl Pts',(83.4200629648173,0.21121934522374,4.07308109263889));
#10232=CARTESIAN_POINT('Ctrl Pts',(83.5875522718362,-3.29979486238722,2.39707260323337));
#10233=CARTESIAN_POINT('Ctrl Pts',(83.7550415788554,-3.80824642224809,-1.46008985560608));
#10234=CARTESIAN_POINT('Ctrl Pts',(83.9225308858744,-0.851483040657149,
-3.98868146515643));
#10235=CARTESIAN_POINT('Ctrl Pts',(84.0900201928935,2.88006522293106,-2.88787595139962));
#10236=CARTESIAN_POINT('Ctrl Pts',(84.2575094999126,3.99097292488117,0.840677293540489));
#10237=CARTESIAN_POINT('Ctrl Pts',(84.4249988069316,1.47039844925099,3.80427806547437));
#10238=CARTESIAN_POINT('Ctrl Pts',(84.5924881139508,-2.38812691276755,3.30627479915456));
#10239=CARTESIAN_POINT('Ctrl Pts',(84.7599774209698,-4.07363820409468,-0.200187365109346));
#10240=CARTESIAN_POINT('Ctrl Pts',(84.9274667279889,-2.05244819362821,-3.52449423484866));
#10241=CARTESIAN_POINT('Ctrl Pts',(85.094956035008,1.83631375377133,-3.64177909773774));
#10242=CARTESIAN_POINT('Ctrl Pts',(85.262445342027,4.05416968532392,-0.445321638380185));
#10243=CARTESIAN_POINT('Ctrl Pts',(85.4299346490461,2.58303918819047,3.15634468195116));
#10244=CARTESIAN_POINT('Ctrl Pts',(85.5974239560652,-1.23846074327946,3.88597712118393));
#10245=CARTESIAN_POINT('Ctrl Pts',(85.7649132630843,-3.93305548107759,1.07966558793672));
#10246=CARTESIAN_POINT('Ctrl Pts',(85.9324025701033,-3.04886851531577,-2.70905961088445));
#10247=CARTESIAN_POINT('Ctrl Pts',(86.0998918771225,0.609557184597477,-4.03274636416857));
#10248=CARTESIAN_POINT('Ctrl Pts',(86.2673811841414,3.71333215303584,-1.68694028354276));
#10249=CARTESIAN_POINT('Ctrl Pts',(86.4348704911607,3.43825695460993,2.19385330254452));
#10250=CARTESIAN_POINT('Ctrl Pts',(86.6023597981796,0.0346291231242072,
4.07840704477139));
#10251=CARTESIAN_POINT('Ctrl Pts',(86.7698491051988,-3.40050857971816,2.25192020246552));
#10252=CARTESIAN_POINT('Ctrl Pts',(86.9373384122178,-3.74144180300417,-1.62364295143421));
#10253=CARTESIAN_POINT('Ctrl Pts',(87.104827719237,-0.677947213373348,-4.02181436355392));
#10254=CARTESIAN_POINT('Ctrl Pts',(87.2723170262559,3.00242783850189,-2.76044023184671));
#10255=CARTESIAN_POINT('Ctrl Pts',(87.4398063332751,3.9508216441462,1.012724807218));
#10256=CARTESIAN_POINT('Ctrl Pts',(87.6072956402942,1.30426788748845,3.86438720584216));
#10257=CARTESIAN_POINT('Ctrl Pts',(87.7747849473132,-2.52907056487011,3.19975081481601));
#10258=CARTESIAN_POINT('Ctrl Pts',(87.9422742543322,-4.06114693025437,-0.376415740761465));
#10259=CARTESIAN_POINT('Ctrl Pts',(88.1097635613515,-1.89788810411,-3.61007256759395));
#10260=CARTESIAN_POINT('Ctrl Pts',(88.2772528683704,1.99230471904383,-3.55883760594312));
#10261=CARTESIAN_POINT('Ctrl Pts',(88.4447421753896,4.06965159818744,-0.269330778730792));
#10262=CARTESIAN_POINT('Ctrl Pts',(88.6122314824086,2.44392468406498,3.26524659676454));
#10263=CARTESIAN_POINT('Ctrl Pts',(88.7797207894276,-1.40558803382318,3.82869762165855));
#10264=CARTESIAN_POINT('Ctrl Pts',(88.9472100964468,-3.97612241986335,0.908324667310112));
#10265=CARTESIAN_POINT('Ctrl Pts',(89.1146994034658,-2.92868745976694,-2.83855473126922));
#10266=CARTESIAN_POINT('Ctrl Pts',(89.2821887104848,0.783630603844815,-4.00256496199248));
#10267=CARTESIAN_POINT('Ctrl Pts',(89.4496780175041,3.78290434825481,-1.52454514234403));
#10268=CARTESIAN_POINT('Ctrl Pts',(89.617167324523,3.34002251362371,2.34069494173511));
#10269=CARTESIAN_POINT('Ctrl Pts',(89.7846566315421,-0.142026075882665,
4.07608044406827));
#10270=CARTESIAN_POINT('Ctrl Pts',(89.9521459385613,-3.49484172472506,2.10254239453794));
#10271=CARTESIAN_POINT('Ctrl Pts',(90.1196352455803,-3.66761690021701,-1.78414951469506));
#10272=CARTESIAN_POINT('Ctrl Pts',(90.2871245525994,-0.503139312267169,
-4.04740089207182));
#10273=CARTESIAN_POINT('Ctrl Pts',(90.4546138596184,3.11915682019817,-2.62782494967201));
#10274=CARTESIAN_POINT('Ctrl Pts',(90.6221031666376,3.90325721534673,1.18287210965676));
#10275=CARTESIAN_POINT('Ctrl Pts',(90.7895924736566,1.13569003616573,3.91724532637939));
#10276=CARTESIAN_POINT('Ctrl Pts',(90.9570817806758,-2.66526874350121,3.08722304209177));
#10277=CARTESIAN_POINT('Ctrl Pts',(91.1245710876948,-4.04103555251424,-0.551938002996637));
#10278=CARTESIAN_POINT('Ctrl Pts',(91.2920603947139,-1.73976677466987,-3.68887676195947));
#10279=CARTESIAN_POINT('Ctrl Pts',(91.4595497017329,2.14455716630937,-3.46921914937233));
#10280=CARTESIAN_POINT('Ctrl Pts',(91.6270390087521,4.07749786226986,-0.0928331999917247));
#10281=CARTESIAN_POINT('Ctrl Pts',(91.7945283157711,2.30022356589825,3.36801906256575));
#10282=CARTESIAN_POINT('Ctrl Pts',(91.9620176227901,-1.57007609244514,3.76423939164203));
#10283=CARTESIAN_POINT('Ctrl Pts',(92.1295069298093,-4.0117323669719,0.735269001609787));
#10284=CARTESIAN_POINT('Ctrl Pts',(92.2969962368283,-2.8030039668561,-2.96270320029105));
#10285=CARTESIAN_POINT('Ctrl Pts',(92.4644855438474,0.956219515839858,-3.96491373724205));
#10286=CARTESIAN_POINT('Ctrl Pts',(92.6319748508664,3.84540632500671,-1.35920972607447));
#10287=CARTESIAN_POINT('Ctrl Pts',(92.7994641578857,3.2354660655269,2.48298752514876));
#10288=CARTESIAN_POINT('Ctrl Pts',(92.9669534649045,-0.318306494350339,
4.06641529905593));
#10289=CARTESIAN_POINT('Ctrl Pts',(93.1344427719238,-3.58283088643105,1.94860893891442));
#10290=CARTESIAN_POINT('Ctrl Pts',(93.3019320789429,-3.58648771117453,-1.94010317901695));
#10291=CARTESIAN_POINT('Ctrl Pts',(93.4694213859618,-0.328237396709569,
-4.06778848006447));
#10292=CARTESIAN_POINT('Ctrl Pts',(93.636910692981,3.23190355653151,-2.48533100535543));
#10293=CARTESIAN_POINT('Ctrl Pts',(93.7485702309937,3.6386515229067,0.0637281040906096));
#10294=CARTESIAN_POINT('Ctrl Pts',(93.8044,3.25944077490411,1.14408268708712));
#10295=CARTESIAN_POINT('Ctrl Pts',(76.2850399531387,-3.44974973462971,0.00177277111675968));
#10296=CARTESIAN_POINT('Ctrl Pts',(76.3185306587644,-3.44656540712918,-0.687240312073141));
#10297=CARTESIAN_POINT('Ctrl Pts',(76.3520213643902,-3.24661788589681,-1.37796575952235));
#10298=CARTESIAN_POINT('Ctrl Pts',(76.3855120700159,-2.86252649231483,-1.94365074249582));
#10299=CARTESIAN_POINT('Ctrl Pts',(76.4413418390223,-2.22223739179093,-2.88666049220702));
#10300=CARTESIAN_POINT('Ctrl Pts',(76.4971716080286,-1.07021892791049,-3.48218717629386));
#10301=CARTESIAN_POINT('Ctrl Pts',(76.553001377035,0.0693892623577064,-3.4593241148768));
#10302=CARTESIAN_POINT('Ctrl Pts',(76.6088311460414,1.20899745262591,-3.43646105345974));
#10303=CARTESIAN_POINT('Ctrl Pts',(76.6646609150477,2.33619536928186,-2.79520824653877));
#10304=CARTESIAN_POINT('Ctrl Pts',(76.7204906840541,2.93815838175754,-1.82729343571165));
#10305=CARTESIAN_POINT('Ctrl Pts',(76.7763204530604,3.54012139423322,-0.859378624884532));
#10306=CARTESIAN_POINT('Ctrl Pts',(76.8321502220668,3.61684950252863,0.435198189848744));
#10307=CARTESIAN_POINT('Ctrl Pts',(76.8879799910732,3.13343047312431,1.46744463563674));
#10308=CARTESIAN_POINT('Ctrl Pts',(76.9438097600795,2.65001144371999,2.49969108142474));
#10309=CARTESIAN_POINT('Ctrl Pts',(76.9996395290858,1.60644527661593,3.26960715826746));
#10310=CARTESIAN_POINT('Ctrl Pts',(77.0554692980922,0.477516896797672,3.42691490934628));
#10311=CARTESIAN_POINT('Ctrl Pts',(77.1112990670986,-0.651411483020579,
3.58422266042509));
#10312=CARTESIAN_POINT('Ctrl Pts',(77.167128836105,-1.86570207555302,3.12892208574002));
#10313=CARTESIAN_POINT('Ctrl Pts',(77.2229586051113,-2.6128997775073,2.26815531216383));
#10314=CARTESIAN_POINT('Ctrl Pts',(77.2630968322316,-3.15008973187288,1.64931606438856));
#10315=CARTESIAN_POINT('Ctrl Pts',(77.3032350593518,-3.44585150244158,0.820901869180171));
#10316=CARTESIAN_POINT('Ctrl Pts',(77.343373286472,-3.45282914603924,-0.00301189592616661));
#10317=CARTESIAN_POINT('Origin',(74.3334724012261,0.,0.));
#10318=CARTESIAN_POINT('',(73.2669448024522,0.,0.));
#10319=CARTESIAN_POINT('',(74.3334724012261,-1.775,-2.17374806848655E-16));
#10320=CARTESIAN_POINT('Origin',(84.65,0.,0.));
#10321=CARTESIAN_POINT('Origin',(94.2,0.,0.));
#10322=CARTESIAN_POINT('',(94.4,-4.05000000000002,4.9598195365468E-16));
#10323=CARTESIAN_POINT('',(94.2,-3.85,-4.71489017671731E-16));
#10324=CARTESIAN_POINT('Origin',(94.4,0.,0.));
#10325=CARTESIAN_POINT('Origin',(9.,6.94,2.5));
#10326=CARTESIAN_POINT('',(13.,7.53615286469164,2.5));
#10327=CARTESIAN_POINT('',(5.,7.53615286469164,2.5));
#10328=CARTESIAN_POINT('',(47.3,7.53615286469164,2.5));
#10329=CARTESIAN_POINT('',(13.,4.94,2.5));
#10330=CARTESIAN_POINT('',(13.,4.94,2.5));
#10331=CARTESIAN_POINT('',(5.,4.94,2.5));
#10332=CARTESIAN_POINT('',(5.,4.94,2.5));
#10333=CARTESIAN_POINT('',(5.,8.94,2.5));
#10334=CARTESIAN_POINT('Origin',(5.,8.94,0.));
#10335=CARTESIAN_POINT('',(5.,7.53615286469164,-2.5));
#10336=CARTESIAN_POINT('Origin',(5.,0.,0.));
#10337=CARTESIAN_POINT('',(5.,4.94,-2.5));
#10338=CARTESIAN_POINT('',(5.,4.94,0.));
#10339=CARTESIAN_POINT('',(5.,8.94,-2.5));
#10340=CARTESIAN_POINT('Origin',(9.,6.94,-2.5));
#10341=CARTESIAN_POINT('',(13.,7.53615286469164,-2.5));
#10342=CARTESIAN_POINT('',(47.3,7.53615286469164,-2.5));
#10343=CARTESIAN_POINT('',(13.,4.94,-2.5));
#10344=CARTESIAN_POINT('',(5.,4.94,-2.5));
#10345=CARTESIAN_POINT('',(13.,4.94,-2.5));
#10346=CARTESIAN_POINT('Origin',(13.,4.94,0.));
#10347=CARTESIAN_POINT('Origin',(13.,0.,0.));
#10348=CARTESIAN_POINT('',(13.,4.94,0.));
#10349=CARTESIAN_POINT('Origin',(5.,4.94,0.));
#10350=CARTESIAN_POINT('Origin',(56.,6.94,2.5));
#10351=CARTESIAN_POINT('',(60.,7.53615286469164,2.5));
#10352=CARTESIAN_POINT('',(52.,7.53615286469164,2.5));
#10353=CARTESIAN_POINT('',(47.3,7.53615286469164,2.5));
#10354=CARTESIAN_POINT('',(60.,4.94,2.5));
#10355=CARTESIAN_POINT('',(60.,4.94,2.5));
#10356=CARTESIAN_POINT('',(52.,4.94,2.5));
#10357=CARTESIAN_POINT('',(52.,4.94,2.5));
#10358=CARTESIAN_POINT('',(52.,8.94,2.5));
#10359=CARTESIAN_POINT('Origin',(52.,8.94,0.));
#10360=CARTESIAN_POINT('',(52.,7.53615286469164,-2.5));
#10361=CARTESIAN_POINT('Origin',(52.,0.,0.));
#10362=CARTESIAN_POINT('',(52.,4.94,-2.5));
#10363=CARTESIAN_POINT('',(52.,4.94,0.));
#10364=CARTESIAN_POINT('',(52.,8.94,-2.5));
#10365=CARTESIAN_POINT('Origin',(56.,6.94,-2.5));
#10366=CARTESIAN_POINT('',(60.,7.53615286469164,-2.5));
#10367=CARTESIAN_POINT('',(47.3,7.53615286469164,-2.5));
#10368=CARTESIAN_POINT('',(60.,4.94,-2.5));
#10369=CARTESIAN_POINT('',(52.,4.94,-2.5));
#10370=CARTESIAN_POINT('',(60.,4.94,-2.5));
#10371=CARTESIAN_POINT('Origin',(60.,4.94,0.));
#10372=CARTESIAN_POINT('Origin',(60.,0.,0.));
#10373=CARTESIAN_POINT('',(60.,4.94,0.));
#10374=CARTESIAN_POINT('Origin',(52.,4.94,0.));
#10375=CARTESIAN_POINT('Origin',(73.6,7.6,0.));
#10376=CARTESIAN_POINT('',(73.6,-7.94,-9.72369558522999E-16));
#10377=CARTESIAN_POINT('Origin',(73.6,0.,0.));
#10378=CARTESIAN_POINT('',(73.6,-7.6,-9.30731567351989E-16));
#10379=CARTESIAN_POINT('Origin',(73.6,0.,0.));
#10380=CARTESIAN_POINT('Origin',(73.05,0.,0.));
#10381=CARTESIAN_POINT('',(72.5,-7.6,-9.30731567351989E-16));
#10382=CARTESIAN_POINT('Origin',(72.5,0.,0.));
#10383=CARTESIAN_POINT('',(73.05,-7.6,-9.30731567351989E-16));
#10384=CARTESIAN_POINT('Origin',(72.5,8.44,0.));
#10385=CARTESIAN_POINT('',(72.5,-7.94,9.72369558522999E-16));
#10386=CARTESIAN_POINT('Origin',(72.5,0.,0.));
#10387=CARTESIAN_POINT('Origin',(47.3,0.,0.));
#10388=CARTESIAN_POINT('',(3.,-7.94,-9.72369558522999E-16));
#10389=CARTESIAN_POINT('',(47.3,-7.94,-9.72369558522999E-16));
#10390=CARTESIAN_POINT('Origin',(3.,0.,0.));
#10391=CARTESIAN_POINT('Origin',(3.,7.6,0.));
#10392=CARTESIAN_POINT('',(3.,-7.6,-9.30731567351989E-16));
#10393=CARTESIAN_POINT('Origin',(3.,0.,0.));
#10394=CARTESIAN_POINT('Origin',(2.45,0.,0.));
#10395=CARTESIAN_POINT('',(1.9,-7.6,-9.30731567351989E-16));
#10396=CARTESIAN_POINT('Origin',(1.9,0.,0.));
#10397=CARTESIAN_POINT('',(2.45,-7.6,-9.30731567351989E-16));
#10398=CARTESIAN_POINT('Origin',(1.9,8.44,0.));
#10399=CARTESIAN_POINT('',(1.9,-7.94,9.72369558522999E-16));
#10400=CARTESIAN_POINT('Origin',(1.9,0.,0.));
#10401=CARTESIAN_POINT('Origin',(47.3,0.,0.));
#10402=CARTESIAN_POINT('',(0.999999999999996,-7.94,-9.72369558522999E-16));
#10403=CARTESIAN_POINT('',(47.3,-7.94,-9.72369558522999E-16));
#10404=CARTESIAN_POINT('Origin',(0.999999999999996,0.,0.));
#10405=CARTESIAN_POINT('Origin',(0.5,7.44,0.));
#10406=CARTESIAN_POINT('',(0.5,-7.44000000000001,-9.11137218565632E-16));
#10407=CARTESIAN_POINT('Origin',(0.500000000000007,0.,0.));
#10408=CARTESIAN_POINT('Origin',(0.749999999999993,0.,0.));
#10409=CARTESIAN_POINT('',(0.749999999999993,-7.69,-9.41753388544315E-16));
#10410=CARTESIAN_POINT('Origin',(47.3,0.,0.));
#10411=CARTESIAN_POINT('',(93.6,-7.94,-9.72369558522999E-16));
#10412=CARTESIAN_POINT('Origin',(93.6,0.,0.));
#10413=CARTESIAN_POINT('',(47.3,-7.94,-9.72369558522999E-16));
#10414=CARTESIAN_POINT('Origin',(94.,0.,0.));
#10415=CARTESIAN_POINT('',(94.4,-7.14,-8.7439781459121E-16));
#10416=CARTESIAN_POINT('Origin',(94.4,0.,0.));
#10417=CARTESIAN_POINT('',(94.,-7.54,-9.23383686557104E-16));
#10418=CARTESIAN_POINT('Origin',(94.4,0.,0.));
#12793=UNCERTAINTY_MEASURE_WITH_UNIT(LENGTH_MEASURE(0.01),#12814,
'DISTANCE_ACCURACY_VALUE',
'Maximum model space distance between geometric entities at asserted c
onnectivities');
#12801=UNCERTAINTY_MEASURE_WITH_UNIT(LENGTH_MEASURE(0.01),#12814,
'DISTANCE_ACCURACY_VALUE',
'Maximum model space distance between geometric entities at asserted c
onnectivities');
#12805=(
GEOMETRIC_REPRESENTATION_CONTEXT(3)
GLOBAL_UNCERTAINTY_ASSIGNED_CONTEXT((#12793))
GLOBAL_UNIT_ASSIGNED_CONTEXT((#12814,#12816,#12817))
REPRESENTATION_CONTEXT('','3D')
);
#12813=(
GEOMETRIC_REPRESENTATION_CONTEXT(3)
GLOBAL_UNCERTAINTY_ASSIGNED_CONTEXT((#12801))
GLOBAL_UNIT_ASSIGNED_CONTEXT((#12814,#12816,#12817))
REPRESENTATION_CONTEXT('','3D')
);
#12814=(
LENGTH_UNIT()
NAMED_UNIT(*)
SI_UNIT(.MILLI.,.METRE.)
);
#12816=(
NAMED_UNIT(*)
PLANE_ANGLE_UNIT()
SI_UNIT($,.RADIAN.)
);
#12817=(
NAMED_UNIT(*)
SI_UNIT($,.STERADIAN.)
SOLID_ANGLE_UNIT()
);
#12821=SHAPE_DEFINITION_REPRESENTATION(#12832,#12856);
#12832=PRODUCT_DEFINITION_SHAPE('',$,#12868);
#12856=SHAPE_REPRESENTATION('',(#4614),#12805);
#12864=PRODUCT_DEFINITION_CONTEXT('part definition',#12899,'design');
#12868=PRODUCT_DEFINITION('2026-10-11-12-17-35-180',
'03_Central_Drive_Shaft_5-8in',#12879,#12864);
#12879=PRODUCT_DEFINITION_FORMATION('',$,#12904);
#12899=APPLICATION_CONTEXT(
'Core Data for Automotive Mechanical Design Process');
#12900=PRODUCT_CONTEXT('part definition',#12899,'mechanical');
#12904=PRODUCT('2026-10-11-12-17-35-180','03_Central_Drive_Shaft_5-8in',
$,(#12900));
#12968=COLOUR_RGB('Grey',0.48,0.52,0.57);
#12969=FILL_AREA_STYLE_COLOUR('',#12968);
#12970=FILL_AREA_STYLE('',(#12969));
#12971=SURFACE_STYLE_FILL_AREA(#12970);
#12972=SURFACE_SIDE_STYLE('',(#12971));
#12973=SURFACE_STYLE_USAGE(.BOTH.,#12972);
#12974=PRESENTATION_STYLE_ASSIGNMENT((#12973));
ENDSEC;
END-ISO-10303-21;
